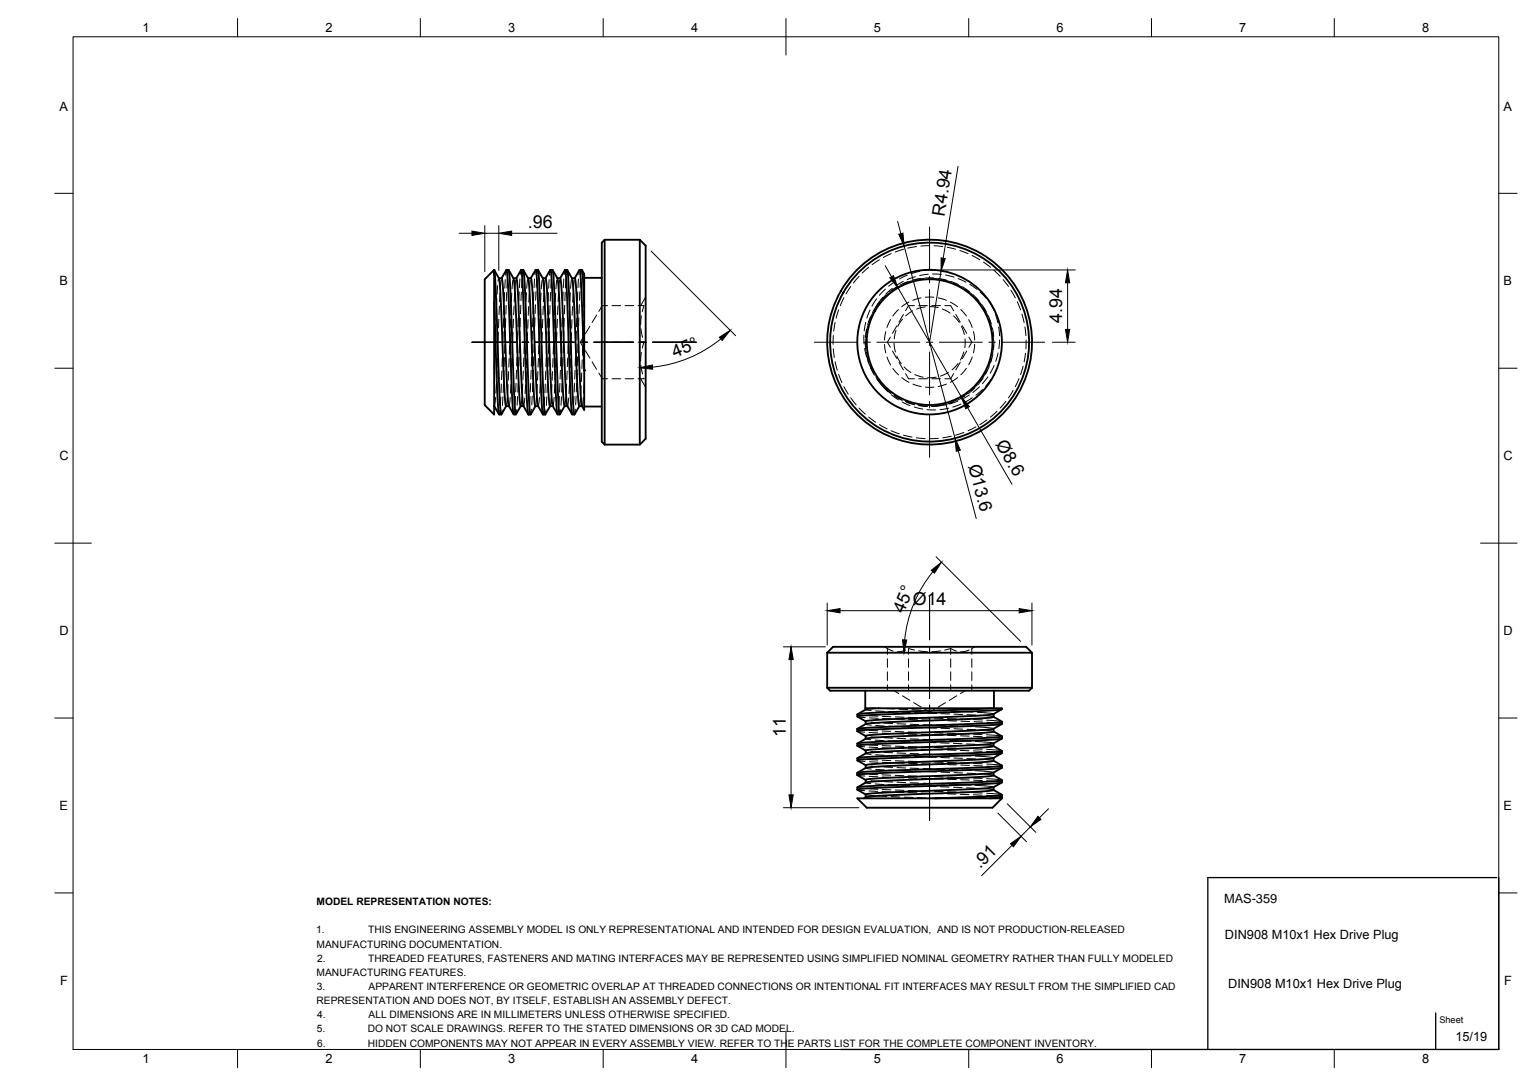
ISO-10303-21;
HEADER;
/* Generated by software containing ST-Developer
 * from STEP Tools, Inc. (www.steptools.com) 
 */

FILE_DESCRIPTION(
/* description */ (''),
/* implementation_level */ '2;1');

FILE_NAME(
/* name */ 'DIN908 M10x1 Hex Drive Plug.step',
/* time_stamp */ '2026-10-15T14:25:16-07:00',
/* author */ (''),
/* organization */ (''),
/* preprocessor_version */ 'ST-DEVELOPER v20.2',
/* originating_system */ 'Autodesk Translation Framework v15.15.0.0',
/* authorisation */ '');

FILE_SCHEMA (('AUTOMOTIVE_DESIGN { 1 0 10303 214 3 1 1 }'));
ENDSEC;

DATA;
#10=MECHANICAL_DESIGN_GEOMETRIC_PRESENTATION_REPRESENTATION('',(#331),#86429);
#254=B_SPLINE_SURFACE_WITH_KNOTS('',3,3,((#65570,#65571,#65572,#65573,#65574,
#65575,#65576,#65577,#65578,#65579,#65580,#65581,#65582,#65583,#65584,#65585,
#65586,#65587,#65588,#65589,#65590,#65591,#65592,#65593,#65594,#65595,#65596,
#65597,#65598,#65599,#65600,#65601,#65602,#65603,#65604,#65605,#65606,#65607,
#65608,#65609,#65610,#65611,#65612,#65613,#65614,#65615),(#65616,#65617,
#65618,#65619,#65620,#65621,#65622,#65623,#65624,#65625,#65626,#65627,#65628,
#65629,#65630,#65631,#65632,#65633,#65634,#65635,#65636,#65637,#65638,#65639,
#65640,#65641,#65642,#65643,#65644,#65645,#65646,#65647,#65648,#65649,#65650,
#65651,#65652,#65653,#65654,#65655,#65656,#65657,#65658,#65659,#65660,#65661),
(#65662,#65663,#65664,#65665,#65666,#65667,#65668,#65669,#65670,#65671,
#65672,#65673,#65674,#65675,#65676,#65677,#65678,#65679,#65680,#65681,#65682,
#65683,#65684,#65685,#65686,#65687,#65688,#65689,#65690,#65691,#65692,#65693,
#65694,#65695,#65696,#65697,#65698,#65699,#65700,#65701,#65702,#65703,#65704,
#65705,#65706,#65707),(#65708,#65709,#65710,#65711,#65712,#65713,#65714,
#65715,#65716,#65717,#65718,#65719,#65720,#65721,#65722,#65723,#65724,#65725,
#65726,#65727,#65728,#65729,#65730,#65731,#65732,#65733,#65734,#65735,#65736,
#65737,#65738,#65739,#65740,#65741,#65742,#65743,#65744,#65745,#65746,#65747,
#65748,#65749,#65750,#65751,#65752,#65753)),.UNSPECIFIED.,.F.,.F.,.F.,(4,
4),(4,1,1,1,1,1,1,1,1,1,1,1,1,1,1,1,1,1,1,1,1,1,1,1,1,1,1,1,1,1,1,1,1,1,
1,1,1,1,1,1,1,1,1,4),(-0.00074044236405861,0.066233565701187),(8.3083844520832,
8.80545257887392,9.30252070566464,10.2966569592461,11.2907932128275,12.284929466409,
13.2790657199904,14.2732019735718,15.2673382271533,16.2614744807347,17.2556107343161,
18.2497469878976,19.243883241479,20.2380194950604,21.2321557486419,22.2262920022233,
23.2204282558048,24.2145645093862,25.2087007629676,26.2028370165491,27.1969732701305,
28.1911095237119,29.1852457772934,30.1793820308748,31.1735182844562,32.1676545380377,
33.1617907916191,34.1559270452005,35.150063298782,36.1441995523634,37.1383358059449,
38.1324720595263,39.1266083131077,40.1207445666892,41.1148808202706,42.109017073852,
43.1031533274335,44.0972895810149,45.0914258345964,46.0855620881778,47.0796983417592,
48.0738345953407,48.5709027221314,49.0687112912862),.UNSPECIFIED.);
#255=B_SPLINE_SURFACE_WITH_KNOTS('',3,3,((#65959,#65960,#65961,#65962,#65963,
#65964,#65965,#65966,#65967,#65968,#65969,#65970,#65971,#65972,#65973,#65974,
#65975,#65976,#65977,#65978,#65979,#65980,#65981,#65982,#65983,#65984,#65985,
#65986,#65987,#65988,#65989,#65990,#65991,#65992,#65993,#65994,#65995,#65996,
#65997,#65998,#65999,#66000,#66001,#66002,#66003,#66004),(#66005,#66006,
#66007,#66008,#66009,#66010,#66011,#66012,#66013,#66014,#66015,#66016,#66017,
#66018,#66019,#66020,#66021,#66022,#66023,#66024,#66025,#66026,#66027,#66028,
#66029,#66030,#66031,#66032,#66033,#66034,#66035,#66036,#66037,#66038,#66039,
#66040,#66041,#66042,#66043,#66044,#66045,#66046,#66047,#66048,#66049,#66050),
(#66051,#66052,#66053,#66054,#66055,#66056,#66057,#66058,#66059,#66060,
#66061,#66062,#66063,#66064,#66065,#66066,#66067,#66068,#66069,#66070,#66071,
#66072,#66073,#66074,#66075,#66076,#66077,#66078,#66079,#66080,#66081,#66082,
#66083,#66084,#66085,#66086,#66087,#66088,#66089,#66090,#66091,#66092,#66093,
#66094,#66095,#66096),(#66097,#66098,#66099,#66100,#66101,#66102,#66103,
#66104,#66105,#66106,#66107,#66108,#66109,#66110,#66111,#66112,#66113,#66114,
#66115,#66116,#66117,#66118,#66119,#66120,#66121,#66122,#66123,#66124,#66125,
#66126,#66127,#66128,#66129,#66130,#66131,#66132,#66133,#66134,#66135,#66136,
#66137,#66138,#66139,#66140,#66141,#66142)),.UNSPECIFIED.,.F.,.F.,.F.,(4,
4),(4,1,1,1,1,1,1,1,1,1,1,1,1,1,1,1,1,1,1,1,1,1,1,1,1,1,1,1,1,1,1,1,1,1,
1,1,1,1,1,1,1,1,1,4),(-0.000415672852192788,0.0663202636511997),(11.6148054166941,
12.112100974609,12.6091691013998,13.6033053549812,14.5974416085626,15.5915778621441,
16.5857141157255,17.5798503693069,18.5739866228884,19.5681228764698,20.5622591300512,
21.5563953836327,22.5505316372141,23.5446678907956,24.538804144377,25.5329403979584,
26.5270766515399,27.5212129051213,28.5153491587027,29.5094854122842,30.5036216658656,
31.497757919447,32.4918941730285,33.4860304266099,34.4801666801914,35.4743029337728,
36.4684391873542,37.4625754409357,38.4567116945171,39.4508479480985,40.44498420168,
41.4391204552614,42.4332567088428,43.4273929624243,44.4215292160057,45.4156654695872,
46.4098017231686,47.40393797675,48.3980742303315,49.3922104839129,50.3863467374943,
51.3804829910758,51.8775511178665,52.3746192446572),.UNSPECIFIED.);
#266=(
BOUNDED_CURVE()
B_SPLINE_CURVE(2,(#66219,#66220,#66221),.UNSPECIFIED.,.F.,.F.)
B_SPLINE_CURVE_WITH_KNOTS((3,3),(-0.639366558443437,-0.433164349146202),
 .UNSPECIFIED.)
CURVE()
GEOMETRIC_REPRESENTATION_ITEM()
RATIONAL_B_SPLINE_CURVE((1.35866716012837,1.4637604307034,1.4637604307034))
REPRESENTATION_ITEM('')
);
#267=(
BOUNDED_CURVE()
B_SPLINE_CURVE(2,(#66223,#66224,#66225),.UNSPECIFIED.,.F.,.F.)
B_SPLINE_CURVE_WITH_KNOTS((3,3),(0.0319010196424348,0.336489692457453),
 .UNSPECIFIED.)
CURVE()
GEOMETRIC_REPRESENTATION_ITEM()
RATIONAL_B_SPLINE_CURVE((1.03712812921102,1.19757240916823,1.03712812921102))
REPRESENTATION_ITEM('')
);
#268=(
BOUNDED_CURVE()
B_SPLINE_CURVE(2,(#66227,#66228,#66229),.UNSPECIFIED.,.F.,.F.)
B_SPLINE_CURVE_WITH_KNOTS((3,3),(0.0319010196424347,0.336489692457453),
 .UNSPECIFIED.)
CURVE()
GEOMETRIC_REPRESENTATION_ITEM()
RATIONAL_B_SPLINE_CURVE((1.03712812921102,1.19757240916823,1.03712812921102))
REPRESENTATION_ITEM('')
);
#269=(
BOUNDED_CURVE()
B_SPLINE_CURVE(2,(#66231,#66232,#66233),.UNSPECIFIED.,.F.,.F.)
B_SPLINE_CURVE_WITH_KNOTS((3,3),(0.0319010196424348,0.336489692457453),
 .UNSPECIFIED.)
CURVE()
GEOMETRIC_REPRESENTATION_ITEM()
RATIONAL_B_SPLINE_CURVE((1.03712812921102,1.19757240916823,1.03712812921102))
REPRESENTATION_ITEM('')
);
#270=(
BOUNDED_CURVE()
B_SPLINE_CURVE(2,(#66235,#66236,#66237),.UNSPECIFIED.,.F.,.F.)
B_SPLINE_CURVE_WITH_KNOTS((3,3),(0.0319010196424349,0.336489692457453),
 .UNSPECIFIED.)
CURVE()
GEOMETRIC_REPRESENTATION_ITEM()
RATIONAL_B_SPLINE_CURVE((1.03712812921102,1.19757240916823,1.03712812921102))
REPRESENTATION_ITEM('')
);
#271=(
BOUNDED_CURVE()
B_SPLINE_CURVE(2,(#66239,#66240,#66241),.UNSPECIFIED.,.F.,.F.)
B_SPLINE_CURVE_WITH_KNOTS((3,3),(0.0319010196424347,0.336489692457453),
 .UNSPECIFIED.)
CURVE()
GEOMETRIC_REPRESENTATION_ITEM()
RATIONAL_B_SPLINE_CURVE((1.03712812921102,1.19757240916823,1.03712812921102))
REPRESENTATION_ITEM('')
);
#272=(
BOUNDED_CURVE()
B_SPLINE_CURVE(2,(#66242,#66243,#66244),.UNSPECIFIED.,.F.,.F.)
B_SPLINE_CURVE_WITH_KNOTS((3,3),(-0.433164349146202,-0.226962139848967),
 .UNSPECIFIED.)
CURVE()
GEOMETRIC_REPRESENTATION_ITEM()
RATIONAL_B_SPLINE_CURVE((1.4637604307034,1.4637604307034,1.35866716012837))
REPRESENTATION_ITEM('')
);
#295=SHAPE_REPRESENTATION_RELATIONSHIP('SRR','None',#86510,#313);
#313=ADVANCED_BREP_SHAPE_REPRESENTATION('',(#349),#86419);
#331=STYLED_ITEM('',(#86609),#349);
#349=MANIFOLD_SOLID_BREP('Body1',#15621);
#898=B_SPLINE_CURVE_WITH_KNOTS('',3,(#63261,#63262,#63263,#63264,#63265,
#63266,#63267,#63268,#63269,#63270,#63271,#63272,#63273,#63274,#63275,#63276,
#63277,#63278,#63279,#63280,#63281,#63282,#63283,#63284,#63285,#63286,#63287,
#63288,#63289,#63290,#63291,#63292,#63293,#63294,#63295,#63296,#63297,#63298,
#63299,#63300,#63301,#63302,#63303,#63304,#63305,#63306,#63307,#63308,#63309,
#63310,#63311,#63312,#63313,#63314,#63315,#63316,#63317,#63318,#63319,#63320,
#63321,#63322,#63323,#63324,#63325,#63326,#63327,#63328,#63329,#63330,#63331,
#63332,#63333,#63334,#63335,#63336,#63337,#63338,#63339),.UNSPECIFIED.,
 .F.,.F.,(4,3,3,3,3,3,3,3,3,3,3,3,3,3,3,3,3,3,3,3,3,3,3,3,3,3,4),(10.3769577827544,
10.5273598900866,10.6774945443399,10.8308192114618,10.9808890436316,11.1358411282296,
11.2907932128275,11.4445181516619,11.5979719285541,11.7512647292242,11.9046292861554,
12.0580308496751,12.211755396569,12.284929466409,12.4385133838143,12.5918292435621,
12.7449877126714,12.8982250015488,13.0515031898628,13.2051123582851,13.2790657199904,
13.432297699739,13.5852451018772,13.7380996304701,13.8908875290217,14.0438933465584,
14.1577916878073),.UNSPECIFIED.);
#899=B_SPLINE_CURVE_WITH_KNOTS('',3,(#63342,#63343,#63344,#63345,#63346,
#63347,#63348,#63349,#63350,#63351,#63352,#63353,#63354,#63355,#63356,#63357,
#63358,#63359,#63360,#63361,#63362,#63363,#63364,#63365,#63366,#63367,#63368,
#63369,#63370,#63371,#63372,#63373,#63374,#63375,#63376,#63377,#63378,#63379,
#63380,#63381,#63382,#63383,#63384,#63385,#63386,#63387,#63388,#63389,#63390,
#63391,#63392,#63393,#63394,#63395,#63396),.UNSPECIFIED.,.F.,.F.,(4,3,3,
3,3,3,3,3,3,3,3,3,3,3,3,3,3,3,4),(11.6150328478183,11.7926764189461,11.9701488858192,
12.112100974609,12.2661530434337,12.4201862996183,12.5744137841679,12.6091691013998,
12.7645204088578,12.919681016886,13.0747528344925,13.2299786470436,13.3852896170894,
13.5409644760237,13.6033053549812,13.7553480979553,13.9070954748021,14.0586995150233,
14.1583240782391),.UNSPECIFIED.);
#900=B_SPLINE_CURVE_WITH_KNOTS('',3,(#63402,#63403,#63404,#63405,#63406,
#63407,#63408,#63409,#63410,#63411,#63412,#63413,#63414,#63415,#63416,#63417,
#63418,#63419,#63420,#63421,#63422,#63423,#63424,#63425,#63426,#63427,#63428,
#63429,#63430,#63431,#63432,#63433,#63434,#63435,#63436,#63437,#63438,#63439,
#63440,#63441,#63442,#63443,#63444,#63445,#63446,#63447,#63448,#63449,#63450,
#63451,#63452,#63453,#63454,#63455,#63456,#63457,#63458,#63459,#63460,#63461,
#63462,#63463,#63464,#63465,#63466,#63467,#63468,#63469,#63470,#63471,#63472,
#63473,#63474,#63475,#63476,#63477,#63478,#63479,#63480,#63481,#63482,#63483,
#63484,#63485,#63486,#63487,#63488,#63489,#63490,#63491,#63492,#63493,#63494,
#63495,#63496,#63497,#63498,#63499,#63500,#63501,#63502,#63503,#63504),
 .UNSPECIFIED.,.F.,.F.,(4,3,3,3,3,3,3,3,3,3,3,3,3,3,3,3,3,3,3,3,3,3,3,3,
3,3,3,3,3,3,3,3,3,3,4),(15.7079632679489,15.8650809592317,16.0223560154779,
16.180095481684,16.2614744807347,16.414856728946,16.5679648062975,16.7209100993148,
16.8739286197668,17.0269845627285,17.1803695780412,17.2556107343161,17.4090275970834,
17.5621709487349,17.7151520567367,17.8682067844267,18.021299206932,18.1747205540646,
18.2497469878976,18.4031557793674,18.5562910052633,18.7092639603358,18.8623105909142,
19.0153949374731,19.1688083680783,19.243883241479,19.3972872546799,19.5504175546535,
19.703385452925,19.8564268889446,20.0095059553496,20.1629140554059,20.2380194950604,
20.3914408227308,20.4420478592521),.UNSPECIFIED.);
#901=B_SPLINE_CURVE_WITH_KNOTS('',3,(#63505,#63506,#63507,#63508,#63509,
#63510,#63511,#63512,#63513,#63514,#63515,#63516,#63517,#63518,#63519,#63520,
#63521,#63522,#63523,#63524,#63525,#63526,#63527,#63528,#63529,#63530,#63531,
#63532,#63533,#63534,#63535,#63536,#63537,#63538),.UNSPECIFIED.,.F.,.F.,
(4,3,3,3,3,3,3,3,3,3,3,4),(14.1577916878073,14.2732019735718,14.4266654812486,
14.5798559651052,14.7328845330507,14.8859866502668,15.039126483985,15.1925945327221,
15.2673382271533,15.4330590962838,15.5979020456747,15.7079632678343),
 .UNSPECIFIED.);
#902=B_SPLINE_CURVE_WITH_KNOTS('',3,(#63540,#63541,#63542,#63543,#63544,
#63545,#63546,#63547,#63548,#63549,#63550,#63551,#63552,#63553,#63554,#63555,
#63556,#63557,#63558,#63559,#63560,#63561,#63562,#63563,#63564,#63565,#63566,
#63567,#63568,#63569,#63570,#63571,#63572,#63573),.UNSPECIFIED.,.F.,.F.,
(4,3,3,3,3,3,3,3,3,3,3,4),(14.1583240782391,14.3099489598577,14.4619231331325,
14.5974416085626,14.7511673052192,14.9046218555822,15.05791544251,15.2112807951612,
15.3646831606929,15.5184085065351,15.5915778621441,15.707963267949),
 .UNSPECIFIED.);
#903=B_SPLINE_CURVE_WITH_KNOTS('',3,(#63574,#63575,#63576,#63577,#63578,
#63579,#63580,#63581,#63582,#63583,#63584,#63585,#63586,#63587,#63588,#63589,
#63590,#63591,#63592,#63593,#63594,#63595,#63596,#63597,#63598,#63599,#63600,
#63601,#63602,#63603,#63604,#63605,#63606,#63607,#63608,#63609,#63610,#63611,
#63612,#63613,#63614,#63615,#63616,#63617,#63618,#63619,#63620,#63621,#63622,
#63623,#63624,#63625,#63626,#63627,#63628,#63629,#63630,#63631,#63632,#63633,
#63634,#63635,#63636,#63637,#63638,#63639,#63640,#63641,#63642,#63643,#63644,
#63645,#63646,#63647,#63648,#63649,#63650,#63651,#63652,#63653,#63654,#63655,
#63656,#63657,#63658,#63659,#63660,#63661,#63662,#63663,#63664,#63665,#63666,
#63667,#63668,#63669,#63670,#63671,#63672,#63673),.UNSPECIFIED.,.F.,.F.,
(4,3,3,3,3,3,3,3,3,3,3,3,3,3,3,3,3,3,3,3,3,3,3,3,3,3,3,3,3,3,3,3,3,4),(15.7079632680668,
15.8594388736004,16.0106884436182,16.1619521092882,16.3132060736808,16.4647924609641,
16.5857141157255,16.7389389348221,16.8918864719011,17.0446686448837,17.1975220592675,
17.3504115327853,17.5036305542145,17.5798503693069,17.733313923022,17.886504454532,
18.0395330715724,18.1926352394518,18.3457751247938,18.4992432258178,18.5739866228884,
18.7274115805076,18.8805635511898,19.033553772357,19.1866182515782,19.3397208031865,
19.4931527076817,19.5681228764698,19.7215125444031,19.8746204229269,20.0276355842012,
20.1805858124463,20.3337471975624,20.4409723240163),.UNSPECIFIED.);
#904=B_SPLINE_CURVE_WITH_KNOTS('',3,(#63679,#63680,#63681,#63682,#63683,
#63684,#63685,#63686,#63687,#63688,#63689,#63690,#63691,#63692,#63693,#63694,
#63695,#63696,#63697,#63698,#63699,#63700,#63701,#63702,#63703,#63704,#63705,
#63706,#63707,#63708,#63709,#63710,#63711,#63712,#63713,#63714,#63715,#63716,
#63717,#63718,#63719,#63720,#63721,#63722,#63723,#63724,#63725,#63726,#63727,
#63728,#63729,#63730,#63731,#63732,#63733,#63734,#63735,#63736,#63737,#63738,
#63739,#63740,#63741,#63742,#63743,#63744,#63745,#63746,#63747,#63748,#63749,
#63750,#63751,#63752,#63753,#63754,#63755,#63756,#63757,#63758,#63759,#63760,
#63761,#63762,#63763,#63764,#63765,#63766,#63767,#63768,#63769,#63770,#63771,
#63772,#63773,#63774,#63775,#63776,#63777,#63778,#63779,#63780,#63781),
 .UNSPECIFIED.,.F.,.F.,(4,3,3,3,3,3,3,3,3,3,3,3,3,3,3,3,3,3,3,3,3,3,3,3,
3,3,3,3,3,3,3,3,3,3,4),(21.99114857526,22.1939267919493,22.2262920022233,
22.3796989418416,22.5328322331403,22.6858031775158,22.838847706263,22.9919298961389,
23.145341118553,23.2204282558048,23.3738358680276,23.5269698461768,23.6799414893234,
23.8329867265599,23.9860696314175,24.13948156771,24.2145645093862,24.3679718714795,
24.5211055961752,24.6740769833984,24.827121964018,24.9802046115219,25.1336162933461,
25.2087007629676,25.3621080840594,25.5152417657962,25.6682131082504,25.8212580418961,
25.9743406411039,26.127752273332,26.2028370165491,26.3562428141984,26.5093760788686,
26.662367028694,26.7245753429587),.UNSPECIFIED.);
#905=B_SPLINE_CURVE_WITH_KNOTS('',3,(#63782,#63783,#63784,#63785,#63786,
#63787,#63788,#63789,#63790,#63791,#63792,#63793,#63794,#63795,#63796,#63797,
#63798,#63799,#63800,#63801,#63802,#63803,#63804,#63805,#63806,#63807,#63808,
#63809,#63810,#63811,#63812,#63813,#63814,#63815),.UNSPECIFIED.,.F.,.F.,
(4,3,3,3,3,3,3,3,3,3,3,4),(20.4420478592521,20.5951172325546,20.7543768615764,
20.9074258209389,21.0605493555233,21.2139862899396,21.2321557486419,21.3836611788031,
21.5355330278844,21.6866431849307,21.8388958800296,21.9911485751285),
 .UNSPECIFIED.);
#906=B_SPLINE_CURVE_WITH_KNOTS('',3,(#63817,#63818,#63819,#63820,#63821,
#63822,#63823,#63824,#63825,#63826,#63827,#63828,#63829,#63830,#63831,#63832,
#63833,#63834,#63835,#63836,#63837,#63838,#63839,#63840,#63841,#63842,#63843,
#63844,#63845,#63846,#63847,#63848,#63849,#63850),.UNSPECIFIED.,.F.,.F.,
(4,3,3,3,3,3,3,3,3,3,3,4),(20.4409723240163,20.5622591300512,20.7156759866491,
20.8688193321945,21.0218004341724,21.1748551560304,21.3279475728055,21.4813689144523,
21.5563953836327,21.7227148730573,21.8881132512756,21.9911485750061),
 .UNSPECIFIED.);
#907=B_SPLINE_CURVE_WITH_KNOTS('',3,(#63851,#63852,#63853,#63854,#63855,
#63856,#63857,#63858,#63859,#63860,#63861,#63862,#63863,#63864,#63865,#63866,
#63867,#63868,#63869,#63870,#63871,#63872,#63873,#63874,#63875,#63876,#63877,
#63878,#63879,#63880,#63881,#63882,#63883,#63884,#63885,#63886,#63887,#63888,
#63889,#63890,#63891,#63892,#63893,#63894,#63895,#63896,#63897,#63898,#63899,
#63900,#63901,#63902,#63903,#63904,#63905,#63906,#63907,#63908,#63909,#63910,
#63911,#63912,#63913,#63914,#63915,#63916,#63917,#63918,#63919,#63920,#63921,
#63922,#63923,#63924,#63925,#63926,#63927,#63928,#63929,#63930,#63931,#63932,
#63933,#63934,#63935,#63936,#63937,#63938,#63939,#63940,#63941,#63942,#63943,
#63944,#63945,#63946,#63947,#63948,#63949,#63950,#63951,#63952,#63953),
 .UNSPECIFIED.,.F.,.F.,(4,3,3,3,3,3,3,3,3,3,3,3,3,3,3,3,3,3,3,3,3,3,3,3,
3,3,3,3,3,3,3,3,3,3,4),(21.9911485751285,22.1479256648879,22.3048452391874,
22.462221546967,22.5505316372141,22.703935658999,22.8570659677062,23.0100338748324,
23.1630753197854,23.3161543951809,23.469562504177,23.5446678907956,23.6980767887443,
23.8512120717938,24.0041850346144,24.1572315981784,24.3103158349244,24.4637290908905,
24.538804144377,24.6922115651092,24.8453453550659,24.9983168139393,25.1513618750143,
25.3044446081105,25.4578563821735,25.5329403979584,25.6863473392698,25.8394806322957,
25.9924515784266,26.145496108951,26.2985783006192,26.4519895248209,26.5270766515399,
26.6804991039507,26.7252324446079),.UNSPECIFIED.);
#908=B_SPLINE_CURVE_WITH_KNOTS('',3,(#63959,#63960,#63961,#63962,#63963,
#63964,#63965,#63966,#63967,#63968,#63969,#63970,#63971,#63972,#63973,#63974,
#63975,#63976,#63977,#63978,#63979,#63980,#63981,#63982,#63983,#63984,#63985,
#63986,#63987,#63988,#63989,#63990,#63991,#63992,#63993,#63994,#63995,#63996,
#63997,#63998,#63999,#64000,#64001,#64002,#64003,#64004,#64005,#64006,#64007,
#64008,#64009,#64010,#64011,#64012,#64013,#64014,#64015,#64016,#64017,#64018,
#64019,#64020,#64021,#64022,#64023,#64024,#64025,#64026,#64027,#64028,#64029,
#64030,#64031,#64032,#64033,#64034,#64035,#64036,#64037,#64038,#64039,#64040,
#64041,#64042,#64043,#64044,#64045,#64046,#64047,#64048,#64049,#64050,#64051,
#64052,#64053,#64054,#64055,#64056,#64057,#64058),.UNSPECIFIED.,.F.,.F.,
(4,3,3,3,3,3,3,3,3,3,3,3,3,3,3,3,3,3,3,3,3,3,3,3,3,3,3,3,3,3,3,3,3,4),(28.2743338824354,
28.4259808413042,28.5773785225841,28.7293453362614,28.8807048174512,29.0329752973723,
29.1852457772934,29.3386531544532,29.4917868936077,29.644758294636,29.7978032879121,
29.9508859474332,30.104297640095,30.1793820308748,30.3327894432698,30.4859232177876,
30.6388946541924,30.7919396824536,30.9450223767831,31.0984341034409,31.1735182844562,
31.3269256011464,31.480059280071,31.6330306212942,31.7860755560757,31.9391581577712,
32.0925697945182,32.1676545380377,32.3210720983193,32.4742063232938,32.6272330512433,
32.7801943527862,32.9333288292476,33.0072870494089),.UNSPECIFIED.);
#909=B_SPLINE_CURVE_WITH_KNOTS('',3,(#64059,#64060,#64061,#64062,#64063,
#64064,#64065,#64066,#64067,#64068,#64069,#64070,#64071,#64072,#64073,#64074,
#64075,#64076,#64077,#64078,#64079,#64080,#64081,#64082,#64083,#64084,#64085,
#64086,#64087,#64088,#64089,#64090,#64091,#64092),.UNSPECIFIED.,.F.,.F.,
(4,3,3,3,3,3,3,3,3,3,3,4),(26.7245753429587,26.8776236986561,27.0372984843933,
27.1969732701305,27.3503806471368,27.5035143861932,27.6564857871786,27.8095307804943,
27.9626134401022,28.1160251329216,28.1911095237119,28.2743338823081),
 .UNSPECIFIED.);
#910=B_SPLINE_CURVE_WITH_KNOTS('',3,(#64094,#64095,#64096,#64097,#64098,
#64099,#64100,#64101,#64102,#64103,#64104,#64105,#64106,#64107,#64108,#64109,
#64110,#64111,#64112,#64113,#64114,#64115,#64116,#64117,#64118,#64119,#64120,
#64121,#64122,#64123,#64124,#64125,#64126,#64127),.UNSPECIFIED.,.F.,.F.,
(4,3,3,3,3,3,3,3,3,3,3,4),(26.7252324446079,26.8783075285994,27.0390338727299,
27.1920808254545,27.3451994950597,27.498632670491,27.5212129051213,27.672785837319,
27.8241164256345,27.9752896314244,28.1265899278275,28.2743338823081),
 .UNSPECIFIED.);
#911=B_SPLINE_CURVE_WITH_KNOTS('',3,(#64128,#64129,#64130,#64131,#64132,
#64133,#64134,#64135,#64136,#64137,#64138,#64139,#64140,#64141,#64142,#64143,
#64144,#64145,#64146,#64147,#64148,#64149,#64150,#64151,#64152,#64153,#64154,
#64155,#64156,#64157,#64158,#64159,#64160,#64161,#64162,#64163,#64164,#64165,
#64166,#64167,#64168,#64169,#64170,#64171,#64172,#64173,#64174,#64175,#64176,
#64177,#64178,#64179,#64180,#64181,#64182,#64183,#64184,#64185,#64186,#64187,
#64188,#64189,#64190,#64191,#64192,#64193,#64194,#64195,#64196,#64197,#64198,
#64199,#64200,#64201,#64202,#64203,#64204,#64205,#64206,#64207,#64208,#64209,
#64210,#64211,#64212,#64213,#64214,#64215,#64216,#64217,#64218,#64219,#64220,
#64221,#64222,#64223,#64224,#64225,#64226,#64227,#64228,#64229,#64230),
 .UNSPECIFIED.,.F.,.F.,(4,3,3,3,3,3,3,3,3,3,3,3,3,3,3,3,3,3,3,3,3,3,3,3,
3,3,3,3,3,3,3,3,3,3,4),(28.2743338824879,28.4750398536421,28.5153491587027,
28.6687564800878,28.8218901621242,28.9748615048833,29.1279064388382,29.2809890383584,
29.4344006708985,29.5094854122842,29.6628928231069,29.8160265965599,29.9689980324053,
30.1220430608655,30.2751257558269,30.4285374837698,30.5036216658656,30.6570290428525,
30.810162781889,30.9631341828541,31.1161791761489,31.2692618357356,31.4226735285337,
31.497757919447,31.651165282527,31.8042990074916,31.9572703942643,32.1103153733462,
32.2633980186889,32.4168096974117,32.4918941730285,32.6453002476881,32.7984336411736,
32.9514213448994,33.0077784099125),.UNSPECIFIED.);
#912=B_SPLINE_CURVE_WITH_KNOTS('',3,(#64236,#64237,#64238,#64239,#64240,
#64241,#64242,#64243,#64244,#64245,#64246,#64247,#64248,#64249,#64250,#64251,
#64252,#64253,#64254,#64255,#64256,#64257,#64258,#64259,#64260,#64261,#64262,
#64263,#64264,#64265,#64266,#64267,#64268,#64269,#64270,#64271,#64272,#64273,
#64274,#64275,#64276,#64277,#64278,#64279,#64280,#64281,#64282,#64283,#64284,
#64285,#64286,#64287,#64288,#64289,#64290,#64291,#64292,#64293,#64294,#64295,
#64296,#64297,#64298,#64299,#64300,#64301,#64302,#64303,#64304,#64305,#64306,
#64307,#64308,#64309,#64310,#64311,#64312,#64313,#64314,#64315,#64316,#64317,
#64318,#64319,#64320,#64321,#64322,#64323,#64324,#64325,#64326,#64327,#64328,
#64329,#64330,#64331,#64332,#64333,#64334,#64335,#64336,#64337,#64338),
 .UNSPECIFIED.,.F.,.F.,(4,3,3,3,3,3,3,3,3,3,3,3,3,3,3,3,3,3,3,3,3,3,3,3,
3,3,3,3,3,3,3,3,3,3,4),(34.5575191894877,34.7128109395726,34.8681775956844,
35.0239713658574,35.150063298782,35.3034707576981,35.456604572422,35.6095760427116,
35.762621095208,35.915703808308,36.0691155452003,36.1441995523634,36.2976084936062,
36.4507438054633,36.6037167826695,36.7567633389953,36.9098475561584,37.0632607739405,
37.1383358059449,37.291739596941,37.4448697549461,37.5978375910733,37.7508790844318,
37.9039582764099,38.0573666045902,38.1324720595263,38.2858811685694,38.4390165973614,
38.5919896412426,38.745036189863,38.8981203569408,39.0515334615024,39.1266083131077,
39.2800571769567,39.2915821620202),.UNSPECIFIED.);
#913=B_SPLINE_CURVE_WITH_KNOTS('',3,(#64339,#64340,#64341,#64342,#64343,
#64344,#64345,#64346,#64347,#64348,#64349,#64350,#64351,#64352,#64353,#64354,
#64355,#64356,#64357,#64358,#64359,#64360,#64361,#64362,#64363,#64364,#64365,
#64366,#64367,#64368,#64369,#64370,#64371,#64372),.UNSPECIFIED.,.F.,.F.,
(4,3,3,3,3,3,3,3,3,3,3,4),(33.0072870494089,33.1617907916191,33.3151984118971,
33.4683323951928,33.6213040405922,33.77434927575,33.9274321760551,34.0808441040777,
34.1559270452005,34.3257930361133,34.4944769778812,34.5575191893185),
 .UNSPECIFIED.);
#914=B_SPLINE_CURVE_WITH_KNOTS('',3,(#64374,#64375,#64376,#64377,#64378,
#64379,#64380,#64381,#64382,#64383,#64384,#64385,#64386,#64387,#64388,#64389,
#64390,#64391,#64392,#64393,#64394,#64395,#64396,#64397,#64398,#64399,#64400,
#64401,#64402,#64403,#64404,#64405,#64406,#64407,#64408,#64409,#64410),
 .UNSPECIFIED.,.F.,.F.,(4,3,3,3,3,3,3,3,3,3,3,3,4),(33.0077784099125,33.1608257171148,
33.3139472904311,33.4673823924497,33.4860304266099,33.6394378388404,33.7925716131929,
33.9455430494321,34.098588077529,34.2516707716947,34.4050824981922,34.4801666801914,
34.5575191894877),.UNSPECIFIED.);
#915=B_SPLINE_CURVE_WITH_KNOTS('',3,(#64411,#64412,#64413,#64414,#64415,
#64416,#64417,#64418,#64419,#64420,#64421,#64422,#64423,#64424,#64425,#64426,
#64427,#64428,#64429,#64430,#64431,#64432,#64433,#64434,#64435,#64436,#64437,
#64438,#64439,#64440,#64441,#64442,#64443,#64444,#64445,#64446,#64447,#64448,
#64449,#64450,#64451,#64452,#64453,#64454,#64455,#64456,#64457,#64458,#64459,
#64460,#64461,#64462,#64463,#64464,#64465,#64466,#64467,#64468,#64469,#64470,
#64471,#64472,#64473,#64474,#64475,#64476,#64477,#64478,#64479,#64480,#64481,
#64482,#64483,#64484,#64485,#64486,#64487,#64488,#64489,#64490,#64491,#64492,
#64493,#64494,#64495,#64496,#64497,#64498,#64499,#64500,#64501,#64502,#64503,
#64504,#64505,#64506,#64507,#64508,#64509,#64510),.UNSPECIFIED.,.F.,.F.,
(4,3,3,3,3,3,3,3,3,3,3,3,3,3,3,3,3,3,3,3,3,3,3,3,3,3,3,3,3,3,3,3,3,4),(34.5575191896116,
34.7092547626843,34.8607382426211,35.014129415409,35.165569538894,35.3199362363334,
35.4743029337728,35.6277102998244,35.7808440270258,35.9338154153095,36.0868603948273,
36.2399430399945,36.3933547176269,36.4684391873542,36.6218468068268,36.7749807893111,
36.9279524338957,37.0809976682432,37.2340805677396,37.3874924949681,37.4625754409357,
37.6159823503777,37.7691156230423,37.9220865602605,38.0751310990094,38.2282133086885,
38.3816245656092,38.4567116945171,38.610129889132,38.7632643739221,38.916288756662,
39.0692475637796,39.2223732435226,39.2904651979605),.UNSPECIFIED.);
#916=B_SPLINE_CURVE_WITH_KNOTS('',3,(#64516,#64517,#64518,#64519,#64520,
#64521,#64522,#64523,#64524,#64525,#64526,#64527,#64528,#64529,#64530,#64531,
#64532,#64533,#64534,#64535,#64536,#64537,#64538,#64539,#64540,#64541,#64542,
#64543,#64544,#64545,#64546,#64547,#64548,#64549,#64550,#64551,#64552,#64553,
#64554,#64555,#64556,#64557,#64558,#64559,#64560,#64561,#64562,#64563,#64564,
#64565,#64566,#64567,#64568,#64569,#64570,#64571,#64572,#64573,#64574,#64575,
#64576,#64577,#64578,#64579,#64580,#64581,#64582,#64583,#64584,#64585,#64586,
#64587,#64588,#64589,#64590,#64591,#64592,#64593,#64594,#64595,#64596,#64597,
#64598,#64599,#64600,#64601,#64602,#64603,#64604,#64605,#64606,#64607,#64608,
#64609,#64610,#64611,#64612,#64613,#64614,#64615,#64616,#64617,#64618),
 .UNSPECIFIED.,.F.,.F.,(4,3,3,3,3,3,3,3,3,3,3,3,3,3,3,3,3,3,3,3,3,3,3,3,
3,3,3,3,3,3,3,3,3,3,4),(40.840704496861,41.0315513197139,41.1148808202706,
41.2683084070192,41.4214620763041,41.5744530701636,41.727516935667,41.8806180818076,
42.0340473903573,42.109017073852,42.2624807464789,42.4156713357008,42.5686999497321,
42.7218020243238,42.8749417647447,43.0284096440709,43.1031533274335,43.256368374023,
43.4093096679249,43.5620891086826,43.714945049858,43.8678400512264,44.021069118693,
44.0972895810149,44.2508939544776,44.404222874785,44.5573870466767,44.7106190333205,
44.8638856297818,45.0174737708723,45.0914258345964,45.2451470488387,45.3985988150857,
45.5518916188261,45.5743044775645),.UNSPECIFIED.);
#917=B_SPLINE_CURVE_WITH_KNOTS('',3,(#64619,#64620,#64621,#64622,#64623,
#64624,#64625,#64626,#64627,#64628,#64629,#64630,#64631,#64632,#64633,#64634,
#64635,#64636,#64637,#64638,#64639,#64640,#64641,#64642,#64643,#64644,#64645,
#64646,#64647,#64648,#64649,#64650,#64651,#64652),.UNSPECIFIED.,.F.,.F.,
(4,3,3,3,3,3,3,3,3,3,3,4),(39.2915821620202,39.4447095027457,39.5976829127759,
39.7507369759808,39.9038361708233,40.0572607936133,40.1207445666892,40.2727807639225,
40.4245502282633,40.5761563774086,40.7278367229112,40.8407044966673),
 .UNSPECIFIED.);
#918=B_SPLINE_CURVE_WITH_KNOTS('',3,(#64654,#64655,#64656,#64657,#64658,
#64659,#64660,#64661,#64662,#64663,#64664,#64665,#64666,#64667,#64668,#64669,
#64670,#64671,#64672,#64673,#64674,#64675,#64676,#64677,#64678,#64679,#64680,
#64681,#64682,#64683,#64684,#64685,#64686,#64687),.UNSPECIFIED.,.F.,.F.,
(4,3,3,3,3,3,3,3,3,3,3,4),(39.2904651979605,39.4508479480985,39.6042568862644,
39.7573921950086,39.910365169076,40.0634117222608,40.2164959362774,40.3699091509537,
40.44498420168,40.6155411212441,40.7848606623605,40.8407044964945),
 .UNSPECIFIED.);
#919=B_SPLINE_CURVE_WITH_KNOTS('',3,(#64688,#64689,#64690,#64691,#64692,
#64693,#64694,#64695,#64696,#64697,#64698,#64699,#64700,#64701,#64702,#64703,
#64704,#64705,#64706,#64707,#64708,#64709,#64710,#64711,#64712,#64713,#64714,
#64715,#64716,#64717,#64718,#64719,#64720,#64721,#64722,#64723,#64724,#64725,
#64726,#64727,#64728,#64729,#64730,#64731,#64732,#64733,#64734,#64735,#64736,
#64737,#64738,#64739,#64740,#64741,#64742,#64743,#64744,#64745,#64746,#64747,
#64748,#64749,#64750,#64751,#64752,#64753,#64754,#64755,#64756,#64757,#64758,
#64759,#64760,#64761,#64762,#64763,#64764,#64765,#64766,#64767,#64768,#64769,
#64770,#64771,#64772,#64773,#64774,#64775,#64776,#64777,#64778,#64779,#64780,
#64781,#64782,#64783,#64784,#64785,#64786,#64787),.UNSPECIFIED.,.F.,.F.,
(4,3,3,3,3,3,3,3,3,3,3,3,3,3,3,3,3,3,3,3,3,3,3,3,3,3,3,3,3,3,3,3,3,4),(40.8407044966673,
40.9957591292645,41.1508780734467,41.3064201957631,41.4391204552614,41.5925295553931,
41.7456649753238,41.8986380104205,42.0516845504698,42.2047687090867,42.3581818054854,
42.4332567088428,42.5866737227815,42.7398171688485,42.8927983148208,43.0458529960652,
43.1989453239065,43.3523665040073,43.4273929624243,43.5807737407789,43.7338808906567,
43.8868257956909,44.0398447353975,44.19290155861,44.3462881466742,44.4215292160057,
44.5749567504601,44.7281103673692,44.8811013089363,45.0341651228667,45.1872662177759,
45.3406954764042,45.4156654695872,45.5747633669549),.UNSPECIFIED.);
#920=B_SPLINE_CURVE_WITH_KNOTS('',3,(#64791,#64792,#64793,#64794,#64795,
#64796,#64797,#64798,#64799,#64800,#64801,#64802,#64803,#64804,#64805,#64806,
#64807,#64808,#64809,#64810,#64811,#64812,#64813,#64814,#64815,#64816,#64817,
#64818,#64819,#64820,#64821,#64822,#64823,#64824,#64825,#64826,#64827,#64828,
#64829,#64830,#64831,#64832,#64833,#64834,#64835,#64836),.UNSPECIFIED.,
 .F.,.F.,(4,3,3,3,3,3,3,3,3,3,3,3,3,3,3,4),(-4.09293042013064,-3.97654501432575,
-3.82746242150663,-3.67863474659495,-3.5299614831974,-3.38122102744219,
-3.23245410916824,-3.08336698099754,-2.98240876074431,-2.83653578429899,
-2.69091995422318,-2.54545308154322,-2.39991629923551,-2.25433443827349,
-2.10845930416463,-2.06815232264671),.UNSPECIFIED.);
#921=B_SPLINE_CURVE_WITH_KNOTS('',3,(#64840,#64841,#64842,#64843,#64844,
#64845,#64846,#64847,#64848,#64849,#64850,#64851,#64852,#64853,#64854,#64855,
#64856,#64857,#64858,#64859,#64860,#64861,#64862,#64863,#64864),
 .UNSPECIFIED.,.F.,.F.,(4,3,3,3,3,3,3,3,4),(4.32144212904479E-15,0.172314051943978,
0.344469545399341,0.497068126790716,0.646463497421989,0.7958397759613,0.945404528325424,
0.994136253581434,1.11639350868616),.UNSPECIFIED.);
#922=B_SPLINE_CURVE_WITH_KNOTS('',3,(#64866,#64867,#64868,#64869,#64870,
#64871,#64872,#64873,#64874,#64875,#64876,#64877,#64878,#64879,#64880,#64881,
#64882,#64883,#64884,#64885,#64886,#64887,#64888,#64889,#64890,#64891,#64892,
#64893,#64894,#64895,#64896,#64897,#64898,#64899,#64900,#64901,#64902,#64903,
#64904,#64905,#64906,#64907,#64908,#64909,#64910,#64911,#64912,#64913,#64914,
#64915,#64916,#64917,#64918,#64919,#64920,#64921,#64922,#64923,#64924,#64925,
#64926,#64927,#64928,#64929,#64930,#64931,#64932,#64933,#64934,#64935,#64936,
#64937,#64938,#64939,#64940,#64941,#64942,#64943,#64944,#64945,#64946,#64947,
#64948,#64949,#64950,#64951,#64952,#64953,#64954,#64955,#64956,#64957,#64958,
#64959,#64960,#64961,#64962,#64963,#64964,#64965,#64966,#64967,#64968,#64969,
#64970,#64971,#64972,#64973,#64974,#64975,#64976,#64977,#64978,#64979,#64980,
#64981,#64982,#64983,#64984,#64985,#64986,#64987,#64988,#64989,#64990,#64991,
#64992,#64993,#64994,#64995,#64996,#64997,#64998),.UNSPECIFIED.,.F.,.F.,
(4,3,3,3,3,3,3,3,3,3,3,3,3,3,3,3,3,3,3,3,3,3,3,3,3,3,3,3,3,3,3,3,3,3,3,
3,3,3,3,3,3,3,3,3,4),(1.11639350886518,1.26540107529424,1.4142593470189,
1.56320326233909,1.71217655620612,1.8615074690152,1.98827250716287,2.13573320085301,
2.28291060830462,2.42991002969188,2.57695920191632,2.72402208004863,2.87141215415248,
2.98240876074431,3.13149538526514,3.28032540437999,3.42899933538523,3.5777379135382,
3.726501525518,3.87558312345145,3.97654501432575,4.1254948724311,4.27419103796277,
4.4227344671354,4.57134929638097,4.71999277787197,4.86896212241735,4.97068126790718,
5.11928286943791,5.26762208690304,5.41580101787194,5.56404404366028,5.71231106677202,
5.86090261216133,5.96481752148862,6.11365060296603,6.26222531479554,6.41064301553827,
6.55912704817221,6.70763670357741,6.85646952638757,6.95895377507006,7.11967437914505,
7.27955756183248,7.39957853315717),.UNSPECIFIED.);
#923=B_SPLINE_CURVE_WITH_KNOTS('',3,(#65000,#65001,#65002,#65003,#65004,
#65005,#65006,#65007,#65008,#65009),.UNSPECIFIED.,.F.,.F.,(4,1,1,1,1,1,
1,4),(7.39957881586575,7.9530900286515,8.94722628223293,9.94136253581436,
10.9354987893958,11.9296350429772,12.9237712965587,13.6827641230453),
 .UNSPECIFIED.);
#924=B_SPLINE_CURVE_WITH_KNOTS('',3,(#65011,#65012,#65013,#65014,#65015,
#65016,#65017,#65018,#65019,#65020,#65021),.UNSPECIFIED.,.F.,.F.,(4,1,1,
1,1,1,1,1,4),(13.6827641230453,13.9179075501401,14.9120438037215,15.906180057303,
16.9003163108844,17.8944525644659,18.8885888180473,19.8827250716287,19.9659494302249),
 .UNSPECIFIED.);
#925=B_SPLINE_CURVE_WITH_KNOTS('',3,(#65023,#65024,#65025,#65026,#65027,
#65028,#65029,#65030,#65031,#65032),.UNSPECIFIED.,.F.,.F.,(4,1,1,1,1,1,
1,4),(19.9659494302249,20.8768613252102,21.8709975787916,22.865133832373,
23.8592700859545,24.8534063395359,25.8475425931173,26.2491347374045),
 .UNSPECIFIED.);
#926=B_SPLINE_CURVE_WITH_KNOTS('',3,(#65034,#65035,#65036,#65037,#65038,
#65039,#65040,#65041,#65042,#65043),.UNSPECIFIED.,.F.,.F.,(4,1,1,1,1,1,
1,4),(26.2491347374045,26.8416788466988,27.8358151002802,28.8299513538617,
29.8240876074431,30.8182238610245,31.812360114606,32.5323200445841),
 .UNSPECIFIED.);
#927=B_SPLINE_CURVE_WITH_KNOTS('',3,(#65045,#65046,#65047,#65048,#65049,
#65050,#65051,#65052,#65053,#65054,#65055,#65056,#65057,#65058,#65059,#65060,
#65061,#65062,#65063,#65064,#65065,#65066,#65067,#65068,#65069,#65070,#65071,
#65072,#65073,#65074,#65075,#65076,#65077,#65078,#65079,#65080,#65081,#65082,
#65083,#65084,#65085,#65086,#65087,#65088,#65089,#65090,#65091,#65092,#65093,
#65094,#65095,#65096,#65097,#65098,#65099,#65100,#65101,#65102,#65103,#65104,
#65105,#65106,#65107,#65108,#65109,#65110,#65111,#65112,#65113,#65114,#65115,
#65116,#65117,#65118,#65119,#65120,#65121,#65122,#65123,#65124,#65125,#65126,
#65127,#65128,#65129,#65130,#65131,#65132,#65133,#65134,#65135,#65136,#65137,
#65138,#65139,#65140,#65141,#65142,#65143,#65144,#65145,#65146,#65147,#65148,
#65149,#65150,#65151,#65152,#65153,#65154,#65155,#65156,#65157,#65158,#65159,
#65160,#65161,#65162,#65163,#65164,#65165,#65166,#65167,#65168,#65169,#65170,
#65171,#65172,#65173,#65174,#65175,#65176,#65177),.UNSPECIFIED.,.F.,.F.,
(4,3,3,3,3,3,3,3,3,3,3,3,3,3,3,3,3,3,3,3,3,3,3,3,3,3,3,3,3,3,3,3,3,3,3,
3,3,3,3,3,3,3,3,3,4),(32.5323201655523,32.7174086039218,32.8064963681874,
32.9552946125721,33.1038336449076,33.2522149461395,33.4006619248636,33.5491341052137,
33.6979294074392,33.8006326217688,33.9494658632194,34.0980406789765,34.246458427882,
34.3949424236234,34.5434519944777,34.6922846579409,34.7947688753503,34.9433609925112,
35.0916940432564,35.2398701083223,35.3881153077529,35.536387325413,35.6849883028127,
35.7889051289317,35.9378748258775,36.0865838740458,36.235133264314,36.3837435031379,
36.5323764787389,36.681326045038,36.7830413825131,36.9321232017769,37.0809501019115,
37.2296225918539,37.3783622855042,37.5271284470279,37.6762148396121,37.7771776360946,
37.9230522499658,38.0686696788295,38.2141381094229,38.3596761871594,38.5052593174765,
38.6511351639275,38.6910128210415),.UNSPECIFIED.);
#928=B_SPLINE_CURVE_WITH_KNOTS('',3,(#65181,#65182,#65183,#65184,#65185,
#65186,#65187,#65188,#65189,#65190),.UNSPECIFIED.,.F.,.F.,(4,1,1,1,1,1,
1,4),(-40.7595863968389,-40.2625182700482,-39.7654501432575,-38.771313889676,
-37.7771776360946,-36.7830413825131,-35.7889051289317,-35.5088569560286),
 .UNSPECIFIED.);
#929=B_SPLINE_CURVE_WITH_KNOTS('',3,(#65192,#65193,#65194,#65195,#65196,
#65197,#65198,#65199,#65200,#65201),.UNSPECIFIED.,.F.,.F.,(4,1,1,1,1,1,
1,4),(-35.5088569560286,-34.7947688753503,-33.8006326217688,-32.8064963681874,
-31.812360114606,-30.8182238610245,-29.8240876074431,-29.225671648849),
 .UNSPECIFIED.);
#930=B_SPLINE_CURVE_WITH_KNOTS('',3,(#65203,#65204,#65205,#65206,#65207,
#65208,#65209,#65210,#65211,#65212),.UNSPECIFIED.,.F.,.F.,(4,1,1,1,1,1,
1,4),(-29.225671648849,-28.8299513538617,-27.8358151002802,-26.8416788466988,
-25.8475425931173,-24.8534063395359,-23.8592700859545,-22.9424863416694),
 .UNSPECIFIED.);
#931=B_SPLINE_CURVE_WITH_KNOTS('',3,(#65214,#65215,#65216,#65217,#65218,
#65219,#65220,#65221,#65222,#65223,#65224),.UNSPECIFIED.,.F.,.F.,(4,1,1,
1,1,1,1,1,4),(-22.9424863416694,-22.8651338323731,-21.8709975787916,-20.8768613252102,
-19.8827250716287,-18.8885888180473,-17.8944525644659,-16.9003163108844,
-16.6593010344898),.UNSPECIFIED.);
#932=B_SPLINE_CURVE_WITH_KNOTS('',3,(#65226,#65227,#65228,#65229,#65230,
#65231,#65232,#65233,#65234,#65235),.UNSPECIFIED.,.F.,.F.,(4,1,1,1,1,1,
1,4),(-16.6593010344898,-15.906180057303,-14.9120438037215,-13.9179075501401,
-12.9237712965587,-11.9296350429772,-10.9354987893958,-10.3761157273102),
 .UNSPECIFIED.);
#933=B_SPLINE_CURVE_WITH_KNOTS('',3,(#65236,#65237,#65238,#65239,#65240,
#65241,#65242,#65243,#65244,#65245,#65246,#65247,#65248,#65249,#65250,#65251,
#65252,#65253,#65254,#65255,#65256,#65257,#65258,#65259,#65260,#65261,#65262,
#65263,#65264,#65265,#65266,#65267,#65268,#65269,#65270,#65271,#65272,#65273,
#65274,#65275,#65276,#65277,#65278,#65279,#65280,#65281,#65282,#65283,#65284,
#65285,#65286,#65287,#65288,#65289,#65290,#65291,#65292,#65293,#65294,#65295,
#65296,#65297,#65298,#65299,#65300,#65301,#65302,#65303,#65304,#65305,#65306,
#65307,#65308,#65309,#65310,#65311,#65312,#65313,#65314,#65315,#65316,#65317,
#65318,#65319,#65320,#65321,#65322,#65323,#65324,#65325,#65326,#65327,#65328,
#65329,#65330,#65331,#65332,#65333,#65334,#65335,#65336,#65337,#65338,#65339,
#65340,#65341,#65342,#65343,#65344,#65345,#65346,#65347,#65348,#65349,#65350,
#65351,#65352,#65353,#65354,#65355,#65356,#65357,#65358,#65359,#65360,#65361,
#65362,#65363,#65364,#65365,#65366,#65367,#65368),.UNSPECIFIED.,.F.,.F.,
(4,3,3,3,3,3,3,3,3,3,3,3,3,3,3,3,3,3,3,3,3,3,3,3,3,3,3,3,3,3,3,3,3,3,3,
3,3,3,3,3,3,3,3,3,4),(-10.3761154186762,-10.2158546220139,-10.0546622936771,
-9.94136253581437,-9.79257454522795,-9.64404543825574,-9.49567371048497,
-9.34723566986522,-9.1987720858116,-9.04998470033248,-8.94722628223293,
-8.79847343390106,-8.64997952782992,-8.50164295391919,-8.35323959238031,
-8.20481047459631,-8.05605665252681,-7.95309002865149,-7.804291834983,-7.65575285344285,
-7.50737160293488,-7.3589246742507,-7.21045254363333,-7.06165728984481,
-6.95895377507006,-6.81012048303958,-6.66154561725903,-6.51312781903422,
-6.36464377561713,-6.21613415793645,-6.06730144977603,-5.96481752148862,
-5.81622542190058,-5.66789238697528,-5.51971633593897,-5.37147114763442,
-5.22319913949464,-5.07459816886151,-4.97068126790718,-4.82366356325693,
-4.67690419063574,-4.53020116852648,-4.3835521535988,-4.23663812113851,
-4.09293042032931),.UNSPECIFIED.);
#934=B_SPLINE_CURVE_WITH_KNOTS('',3,(#65371,#65372,#65373,#65374,#65375,
#65376,#65377,#65378,#65379,#65380,#65381,#65382,#65383,#65384,#65385,#65386,
#65387,#65388,#65389,#65390,#65391,#65392,#65393,#65394,#65395,#65396,#65397,
#65398,#65399,#65400,#65401,#65402,#65403,#65404),.UNSPECIFIED.,.F.,.F.,
(4,3,3,3,3,3,3,3,3,3,3,4),(45.5747633669549,45.7279460916964,45.8809709137411,
46.0340726659095,46.1872157257738,46.3406852415556,46.4098017231686,46.5617942570585,
46.7135157473756,46.8650726102834,47.0166960136029,47.1238898038469),
 .UNSPECIFIED.);
#935=B_SPLINE_CURVE_WITH_KNOTS('',3,(#65406,#65407,#65408,#65409,#65410,
#65411,#65412,#65413,#65414,#65415,#65416,#65417,#65418,#65419,#65420,#65421,
#65422,#65423,#65424,#65425,#65426,#65427,#65428,#65429,#65430,#65431,#65432,
#65433,#65434,#65435,#65436,#65437,#65438,#65439,#65440,#65441,#65442,#65443,
#65444,#65445,#65446,#65447,#65448,#65449,#65450,#65451,#65452,#65453,#65454,
#65455,#65456,#65457,#65458,#65459,#65460,#65461,#65462,#65463,#65464,#65465,
#65466,#65467,#65468,#65469,#65470,#65471,#65472),.UNSPECIFIED.,.F.,.F.,
(4,3,3,3,3,3,3,3,3,3,3,3,3,3,3,3,3,3,3,3,3,3,4),(47.1238898040689,47.3128509909798,
47.40393797675,47.5575421867538,47.710870940444,47.8640349431444,48.0172667587525,
48.1705331829181,48.3241211524605,48.3980742303315,48.5517950120318,48.7052464258146,
48.8585386455141,49.0119052759824,49.1653104318385,49.3190408342028,49.3922104839129,
49.5426217757813,49.692761485266,49.8462863076115,49.9963515219788,50.1516061483134,
50.306860774648),.UNSPECIFIED.);
#936=B_SPLINE_CURVE_WITH_KNOTS('',3,(#65476,#65477,#65478,#65479,#65480,
#65481,#65482,#65483,#65484,#65485,#65486,#65487,#65488,#65489,#65490,#65491,
#65492,#65493,#65494,#65495,#65496,#65497,#65498,#65499,#65500,#65501,#65502,
#65503,#65504,#65505,#65506,#65507,#65508,#65509,#65510,#65511,#65512,#65513,
#65514,#65515,#65516,#65517,#65518),.UNSPECIFIED.,.F.,.F.,(4,3,3,3,3,3,
3,3,3,3,3,3,3,3,4),(47.1238898040128,47.2782816278034,47.4323697908821,
47.5927359919967,47.7466225144832,47.9005181633557,48.054632188318,48.0738345953407,
48.2280558285865,48.382092629286,48.5360906232682,48.5709027221314,48.7482748367486,
48.9259950495598,49.0679708489221),.UNSPECIFIED.);
#937=B_SPLINE_CURVE_WITH_KNOTS('',3,(#65519,#65520,#65521,#65522,#65523,
#65524,#65525,#65526,#65527,#65528,#65529,#65530,#65531,#65532,#65533,#65534,
#65535,#65536,#65537,#65538,#65539,#65540,#65541,#65542,#65543,#65544,#65545,
#65546,#65547,#65548,#65549,#65550,#65551,#65552,#65553,#65554,#65555),
 .UNSPECIFIED.,.F.,.F.,(4,3,3,3,3,3,3,3,3,3,3,3,4),(45.5743044775645,45.7276698135094,
45.8810880641648,46.0348251362156,46.0855620881778,46.2375386974501,46.3892415635035,
46.5407859647282,46.6924252089547,46.8441117319342,46.9961635381894,47.0796983417592,
47.1238898038469),.UNSPECIFIED.);
#938=B_SPLINE_CURVE_WITH_KNOTS('',3,(#65558,#65559,#65560,#65561),
 .UNSPECIFIED.,.F.,.F.,(4,4),(-0.968477696161942,-0.935071686684093),
 .UNSPECIFIED.);
#939=B_SPLINE_CURVE_WITH_KNOTS('',3,(#65564,#65565,#65566,#65567,#65568,
#65569),.UNSPECIFIED.,.F.,.F.,(4,2,4),(8.52351753051953E-6,0.0223434875386195,
0.0446411083741544),.UNSPECIFIED.);
#940=B_SPLINE_CURVE_WITH_KNOTS('',3,(#65755,#65756,#65757,#65758),
 .UNSPECIFIED.,.F.,.F.,(4,4),(0.,0.000836946426958433),.UNSPECIFIED.);
#941=B_SPLINE_CURVE_WITH_KNOTS('',3,(#65759,#65760,#65761,#65762,#65763,
#65764,#65765,#65766,#65767,#65768,#65769,#65770,#65771,#65772,#65773,#65774,
#65775,#65776,#65777,#65778,#65779,#65780,#65781,#65782,#65783,#65784,#65785,
#65786,#65787,#65788,#65789,#65790,#65791,#65792,#65793,#65794,#65795,#65796,
#65797,#65798,#65799,#65800,#65801,#65802,#65803,#65804,#65805,#65806,#65807,
#65808,#65809,#65810,#65811,#65812,#65813,#65814,#65815,#65816,#65817,#65818,
#65819,#65820,#65821,#65822,#65823,#65824,#65825),.UNSPECIFIED.,.F.,.F.,
(4,3,3,3,3,3,3,3,3,3,3,3,3,3,3,3,3,3,3,3,3,3,4),(0.,0.0393121242914099,
0.117107898720596,0.167166306519262,0.189098627719502,0.208304762061158,
0.258210465370092,0.32305163930505,0.355694799905693,0.380210492454201,
0.409081485034023,0.483065857864488,0.517575161109925,0.554598739699055,
0.575971627854233,0.64977279486791,0.698159307576866,0.728055674524275,
0.746545820285823,0.819560974564155,0.852041521246935,0.875301939868949,
0.922805662986717),.UNSPECIFIED.);
#942=B_SPLINE_CURVE_WITH_KNOTS('',3,(#65826,#65827,#65828,#65829,#65830,
#65831,#65832,#65833,#65834,#65835,#65836,#65837,#65838,#65839,#65840,#65841,
#65842,#65843,#65844,#65845,#65846,#65847,#65848,#65849,#65850,#65851,#65852,
#65853,#65854,#65855,#65856,#65857,#65858,#65859,#65860,#65861,#65862,#65863,
#65864,#65865,#65866,#65867,#65868,#65869,#65870,#65871,#65872,#65873,#65874,
#65875,#65876,#65877,#65878,#65879,#65880,#65881,#65882,#65883,#65884,#65885,
#65886,#65887,#65888,#65889),.UNSPECIFIED.,.F.,.F.,(4,3,3,3,3,3,3,3,3,3,
3,3,3,3,3,3,3,3,3,3,3,4),(-0.968477696161958,-0.93346935475494,-0.87462218483068,
-0.838968787568558,-0.787473146091247,-0.753349378601184,-0.721529105370558,
-0.646900128137883,-0.59677334563425,-0.567483204022971,-0.543548087950493,
-0.480303919736905,-0.421085426012196,-0.392827821972742,-0.362136007930906,
-0.285930318294375,-0.243429944838067,-0.203365840094899,-0.175996194930052,
-0.0982285541899456,-0.0209966080041514,-2.23186798271618E-15),
 .UNSPECIFIED.);
#943=B_SPLINE_CURVE_WITH_KNOTS('',3,(#65895,#65896,#65897,#65898,#65899,
#65900,#65901,#65902,#65903,#65904,#65905,#65906,#65907,#65908,#65909,#65910,
#65911,#65912,#65913,#65914,#65915,#65916,#65917,#65918,#65919,#65920,#65921,
#65922,#65923,#65924,#65925,#65926,#65927,#65928,#65929,#65930,#65931,#65932,
#65933,#65934,#65935,#65936,#65937,#65938,#65939,#65940,#65941,#65942,#65943,
#65944,#65945,#65946,#65947,#65948,#65949,#65950,#65951,#65952,#65953,#65954,
#65955,#65956,#65957,#65958),.UNSPECIFIED.,.F.,.F.,(4,3,3,3,3,3,3,3,3,3,
3,3,3,3,3,3,3,3,3,3,3,4),(-0.953001334118943,-0.926795214108053,-0.867226959656485,
-0.843238497088046,-0.822042260146921,-0.745112575774413,-0.716203876023601,
-0.693609567103274,-0.617312067174212,-0.566983454838404,-0.537479678376499,
-0.514261574452167,-0.450249178495506,-0.393119621046725,-0.34952529407956,
-0.293393258181454,-0.221730948700384,-0.182710666717766,-0.157793989938048,
-0.085628124075386,-0.0150794994075627,-1.37622244676669E-15),
 .UNSPECIFIED.);
#944=B_SPLINE_CURVE_WITH_KNOTS('',3,(#66144,#66145,#66146,#66147),
 .UNSPECIFIED.,.F.,.F.,(4,4),(0.,0.0112420344023245),.UNSPECIFIED.);
#945=B_SPLINE_CURVE_WITH_KNOTS('',3,(#66148,#66149,#66150,#66151),
 .UNSPECIFIED.,.F.,.F.,(4,4),(0.,0.0131288794431488),.UNSPECIFIED.);
#946=B_SPLINE_CURVE_WITH_KNOTS('',3,(#66152,#66153,#66154,#66155,#66156,
#66157,#66158,#66159,#66160,#66161,#66162,#66163,#66164,#66165,#66166,#66167,
#66168,#66169,#66170,#66171,#66172,#66173,#66174,#66175,#66176,#66177,#66178,
#66179,#66180,#66181,#66182,#66183,#66184,#66185,#66186,#66187,#66188,#66189,
#66190,#66191,#66192,#66193,#66194,#66195,#66196,#66197,#66198,#66199,#66200,
#66201,#66202,#66203,#66204,#66205,#66206,#66207,#66208,#66209,#66210,#66211,
#66212,#66213,#66214,#66215),.UNSPECIFIED.,.F.,.F.,(4,3,3,3,3,3,3,3,3,3,
3,3,3,3,3,3,3,3,3,3,3,4),(0.0447297051812948,0.11579384797572,0.169972513625885,
0.195080510370564,0.269055930443271,0.323648223080396,0.345181704722379,
0.365728274421021,0.407621329269858,0.482026226691156,0.487425100991772,
0.524760575111112,0.54632412226274,0.620775662398705,0.672151363956664,
0.703230969871393,0.723527065514623,0.784142853240842,0.821242619777157,
0.858091484337553,0.935825551512836,0.965990216419499),.UNSPECIFIED.);
#1309=CONICAL_SURFACE('',#16920,0.320138837486628,1.0471975511966);
#1310=CONICAL_SURFACE('',#16925,0.1225,1.0267507402002);
#1311=CONICAL_SURFACE('',#16933,0.465,0.785398163397448);
#1312=CONICAL_SURFACE('',#16941,0.69,0.785398163397449);
#1313=CONICAL_SURFACE('',#16945,0.68,0.785398163397449);
#1520=CYLINDRICAL_SURFACE('',#16903,0.4372);
#1521=CYLINDRICAL_SURFACE('',#16905,0.4372);
#1522=CYLINDRICAL_SURFACE('',#16906,0.4372);
#1523=CYLINDRICAL_SURFACE('',#16907,0.4372);
#1524=CYLINDRICAL_SURFACE('',#16908,0.4372);
#1525=CYLINDRICAL_SURFACE('',#16909,0.4372);
#1526=CYLINDRICAL_SURFACE('',#16910,0.4942);
#1527=CYLINDRICAL_SURFACE('',#16913,0.4372);
#1528=CYLINDRICAL_SURFACE('',#16937,0.44);
#1529=CYLINDRICAL_SURFACE('',#16943,0.7);
#1718=FACE_BOUND('',#4064,.T.);
#1719=FACE_BOUND('',#4070,.T.);
#1720=FACE_BOUND('',#4075,.T.);
#2236=CIRCLE('',#16904,0.4372);
#2237=CIRCLE('',#16911,0.4942);
#2238=CIRCLE('',#16912,0.4942);
#2239=CIRCLE('',#16914,0.4372);
#2240=CIRCLE('',#16916,0.44);
#2241=CIRCLE('',#16918,0.4942);
#2242=CIRCLE('',#16919,0.4942);
#2243=CIRCLE('',#16921,0.308675134594813);
#2244=CIRCLE('',#16926,0.243346949651439);
#2245=CIRCLE('',#16932,0.43);
#2246=CIRCLE('',#16935,0.44);
#2247=CIRCLE('',#16936,0.44);
#2248=CIRCLE('',#16938,0.44);
#2249=CIRCLE('',#16940,0.68);
#2250=CIRCLE('',#16942,0.7);
#2251=CIRCLE('',#16944,0.7);
#2252=CIRCLE('',#16946,0.66);
#3055=FACE_OUTER_BOUND('',#4043,.T.);
#3056=FACE_OUTER_BOUND('',#4044,.T.);
#3057=FACE_OUTER_BOUND('',#4045,.T.);
#3058=FACE_OUTER_BOUND('',#4046,.T.);
#3059=FACE_OUTER_BOUND('',#4047,.T.);
#3060=FACE_OUTER_BOUND('',#4048,.T.);
#3061=FACE_OUTER_BOUND('',#4049,.T.);
#3062=FACE_OUTER_BOUND('',#4050,.T.);
#3063=FACE_OUTER_BOUND('',#4051,.T.);
#3064=FACE_OUTER_BOUND('',#4052,.T.);
#3065=FACE_OUTER_BOUND('',#4053,.T.);
#3066=FACE_OUTER_BOUND('',#4054,.T.);
#3067=FACE_OUTER_BOUND('',#4055,.T.);
#3068=FACE_OUTER_BOUND('',#4056,.T.);
#3069=FACE_OUTER_BOUND('',#4057,.T.);
#3070=FACE_OUTER_BOUND('',#4058,.T.);
#3071=FACE_OUTER_BOUND('',#4059,.T.);
#3072=FACE_OUTER_BOUND('',#4060,.T.);
#3073=FACE_OUTER_BOUND('',#4061,.T.);
#3074=FACE_OUTER_BOUND('',#4062,.T.);
#3075=FACE_OUTER_BOUND('',#4063,.T.);
#3076=FACE_OUTER_BOUND('',#4065,.T.);
#3077=FACE_OUTER_BOUND('',#4066,.T.);
#3078=FACE_OUTER_BOUND('',#4067,.T.);
#3079=FACE_OUTER_BOUND('',#4068,.T.);
#3080=FACE_OUTER_BOUND('',#4069,.T.);
#3081=FACE_OUTER_BOUND('',#4071,.T.);
#3082=FACE_OUTER_BOUND('',#4072,.T.);
#3083=FACE_OUTER_BOUND('',#4073,.T.);
#3084=FACE_OUTER_BOUND('',#4074,.T.);
#4043=EDGE_LOOP('',(#13305,#13306,#13307,#13308));
#4044=EDGE_LOOP('',(#13309,#13310,#13311,#13312,#13313,#13314));
#4045=EDGE_LOOP('',(#13315,#13316,#13317,#13318,#13319,#13320));
#4046=EDGE_LOOP('',(#13321,#13322,#13323,#13324,#13325,#13326));
#4047=EDGE_LOOP('',(#13327,#13328,#13329,#13330,#13331,#13332));
#4048=EDGE_LOOP('',(#13333,#13334,#13335,#13336,#13337,#13338));
#4049=EDGE_LOOP('',(#13339,#13340,#13341,#13342,#13343,#13344,#13345,#13346,
#13347,#13348,#13349,#13350,#13351,#13352,#13353,#13354));
#4050=EDGE_LOOP('',(#13355,#13356,#13357,#13358,#13359,#13360));
#4051=EDGE_LOOP('',(#13361,#13362,#13363,#13364));
#4052=EDGE_LOOP('',(#13365,#13366,#13367,#13368,#13369,#13370,#13371,#13372,
#13373,#13374,#13375,#13376,#13377,#13378,#13379,#13380,#13381,#13382,#13383,
#13384,#13385,#13386,#13387,#13388));
#4053=EDGE_LOOP('',(#13389,#13390,#13391,#13392,#13393));
#4054=EDGE_LOOP('',(#13394,#13395,#13396,#13397,#13398,#13399,#13400,#13401,
#13402,#13403,#13404,#13405,#13406,#13407,#13408,#13409,#13410,#13411,#13412,
#13413,#13414,#13415,#13416,#13417,#13418));
#4055=EDGE_LOOP('',(#13419,#13420,#13421,#13422,#13423,#13424,#13425,#13426,
#13427,#13428));
#4056=EDGE_LOOP('',(#13429,#13430,#13431,#13432));
#4057=EDGE_LOOP('',(#13433,#13434,#13435,#13436));
#4058=EDGE_LOOP('',(#13437,#13438,#13439,#13440));
#4059=EDGE_LOOP('',(#13441,#13442,#13443));
#4060=EDGE_LOOP('',(#13444,#13445,#13446,#13447));
#4061=EDGE_LOOP('',(#13448,#13449,#13450,#13451));
#4062=EDGE_LOOP('',(#13452,#13453,#13454,#13455,#13456));
#4063=EDGE_LOOP('',(#13457,#13458,#13459,#13460,#13461,#13462));
#4064=EDGE_LOOP('',(#13463));
#4065=EDGE_LOOP('',(#13464));
#4066=EDGE_LOOP('',(#13465,#13466,#13467,#13468,#13469,#13470,#13471));
#4067=EDGE_LOOP('',(#13472,#13473,#13474,#13475,#13476));
#4068=EDGE_LOOP('',(#13477,#13478,#13479,#13480,#13481,#13482,#13483,#13484));
#4069=EDGE_LOOP('',(#13485));
#4070=EDGE_LOOP('',(#13486));
#4071=EDGE_LOOP('',(#13487,#13488,#13489,#13490));
#4072=EDGE_LOOP('',(#13491,#13492,#13493,#13494));
#4073=EDGE_LOOP('',(#13495,#13496,#13497,#13498));
#4074=EDGE_LOOP('',(#13499));
#4075=EDGE_LOOP('',(#13500));
#4981=LINE('',#63259,#5841);
#4982=LINE('',#63400,#5842);
#4983=LINE('',#63677,#5843);
#4984=LINE('',#63957,#5844);
#4985=LINE('',#64234,#5845);
#4986=LINE('',#64514,#5846);
#4987=LINE('',#66246,#5847);
#4988=LINE('',#66250,#5848);
#4989=LINE('',#66252,#5849);
#4990=LINE('',#66253,#5850);
#4991=LINE('',#66256,#5851);
#4992=LINE('',#66257,#5852);
#4993=LINE('',#66260,#5853);
#4994=LINE('',#66261,#5854);
#4995=LINE('',#66265,#5855);
#4996=LINE('',#66269,#5856);
#4997=LINE('',#66270,#5857);
#4998=LINE('',#66273,#5858);
#4999=LINE('',#66274,#5859);
#5000=LINE('',#66276,#5860);
#5001=LINE('',#66282,#5861);
#5002=LINE('',#66290,#5862);
#5003=LINE('',#66297,#5863);
#5004=LINE('',#66301,#5864);
#5005=LINE('',#66304,#5865);
#5841=VECTOR('',#20134,0.4372);
#5842=VECTOR('',#20139,0.4372);
#5843=VECTOR('',#20142,0.4372);
#5844=VECTOR('',#20145,0.4372);
#5845=VECTOR('',#20148,0.4372);
#5846=VECTOR('',#20151,0.4372);
#5847=VECTOR('',#20174,0.320138837486628);
#5848=VECTOR('',#20179,1.);
#5849=VECTOR('',#20180,1.);
#5850=VECTOR('',#20181,1.);
#5851=VECTOR('',#20184,1.);
#5852=VECTOR('',#20185,1.);
#5853=VECTOR('',#20188,1.);
#5854=VECTOR('',#20189,1.);
#5855=VECTOR('',#20192,0.1225);
#5856=VECTOR('',#20197,1.);
#5857=VECTOR('',#20198,1.);
#5858=VECTOR('',#20201,1.);
#5859=VECTOR('',#20202,1.);
#5860=VECTOR('',#20205,1.);
#5861=VECTOR('',#20214,0.465);
#5862=VECTOR('',#20225,0.44);
#5863=VECTOR('',#20234,0.69);
#5864=VECTOR('',#20239,0.7);
#5865=VECTOR('',#20242,0.68);
#7128=VERTEX_POINT('',#63257);
#7129=VERTEX_POINT('',#63258);
#7130=VERTEX_POINT('',#63260);
#7131=VERTEX_POINT('',#63340);
#7132=VERTEX_POINT('',#63398);
#7133=VERTEX_POINT('',#63399);
#7134=VERTEX_POINT('',#63401);
#7135=VERTEX_POINT('',#63539);
#7136=VERTEX_POINT('',#63675);
#7137=VERTEX_POINT('',#63676);
#7138=VERTEX_POINT('',#63678);
#7139=VERTEX_POINT('',#63816);
#7140=VERTEX_POINT('',#63955);
#7141=VERTEX_POINT('',#63956);
#7142=VERTEX_POINT('',#63958);
#7143=VERTEX_POINT('',#64093);
#7144=VERTEX_POINT('',#64232);
#7145=VERTEX_POINT('',#64233);
#7146=VERTEX_POINT('',#64235);
#7147=VERTEX_POINT('',#64373);
#7148=VERTEX_POINT('',#64512);
#7149=VERTEX_POINT('',#64513);
#7150=VERTEX_POINT('',#64515);
#7151=VERTEX_POINT('',#64653);
#7152=VERTEX_POINT('',#64789);
#7153=VERTEX_POINT('',#64790);
#7154=VERTEX_POINT('',#64837);
#7155=VERTEX_POINT('',#64839);
#7156=VERTEX_POINT('',#64865);
#7157=VERTEX_POINT('',#64999);
#7158=VERTEX_POINT('',#65010);
#7159=VERTEX_POINT('',#65022);
#7160=VERTEX_POINT('',#65033);
#7161=VERTEX_POINT('',#65044);
#7162=VERTEX_POINT('',#65178);
#7163=VERTEX_POINT('',#65180);
#7164=VERTEX_POINT('',#65191);
#7165=VERTEX_POINT('',#65202);
#7166=VERTEX_POINT('',#65213);
#7167=VERTEX_POINT('',#65225);
#7168=VERTEX_POINT('',#65370);
#7169=VERTEX_POINT('',#65405);
#7170=VERTEX_POINT('',#65473);
#7171=VERTEX_POINT('',#65475);
#7172=VERTEX_POINT('',#65557);
#7173=VERTEX_POINT('',#65562);
#7174=VERTEX_POINT('',#65754);
#7175=VERTEX_POINT('',#65891);
#7176=VERTEX_POINT('',#65893);
#7177=VERTEX_POINT('',#66143);
#7178=VERTEX_POINT('',#66217);
#7179=VERTEX_POINT('',#66218);
#7180=VERTEX_POINT('',#66222);
#7181=VERTEX_POINT('',#66226);
#7182=VERTEX_POINT('',#66230);
#7183=VERTEX_POINT('',#66234);
#7184=VERTEX_POINT('',#66238);
#7185=VERTEX_POINT('',#66245);
#7186=VERTEX_POINT('',#66249);
#7187=VERTEX_POINT('',#66251);
#7188=VERTEX_POINT('',#66255);
#7189=VERTEX_POINT('',#66259);
#7190=VERTEX_POINT('',#66263);
#7191=VERTEX_POINT('',#66264);
#7192=VERTEX_POINT('',#66268);
#7193=VERTEX_POINT('',#66272);
#7194=VERTEX_POINT('',#66279);
#7195=VERTEX_POINT('',#66284);
#7196=VERTEX_POINT('',#66288);
#7197=VERTEX_POINT('',#66292);
#7198=VERTEX_POINT('',#66295);
#7199=VERTEX_POINT('',#66299);
#7200=VERTEX_POINT('',#66303);
#9274=EDGE_CURVE('',#7128,#7129,#4981,.T.);
#9275=EDGE_CURVE('',#7130,#7128,#898,.T.);
#9276=EDGE_CURVE('',#7131,#7130,#2236,.T.);
#9277=EDGE_CURVE('',#7131,#7129,#899,.T.);
#9278=EDGE_CURVE('',#7132,#7133,#4982,.T.);
#9279=EDGE_CURVE('',#7134,#7132,#900,.T.);
#9280=EDGE_CURVE('',#7128,#7134,#901,.T.);
#9281=EDGE_CURVE('',#7129,#7135,#902,.T.);
#9282=EDGE_CURVE('',#7135,#7133,#903,.T.);
#9283=EDGE_CURVE('',#7136,#7137,#4983,.T.);
#9284=EDGE_CURVE('',#7138,#7136,#904,.T.);
#9285=EDGE_CURVE('',#7132,#7138,#905,.T.);
#9286=EDGE_CURVE('',#7133,#7139,#906,.T.);
#9287=EDGE_CURVE('',#7139,#7137,#907,.T.);
#9288=EDGE_CURVE('',#7140,#7141,#4984,.T.);
#9289=EDGE_CURVE('',#7142,#7140,#908,.T.);
#9290=EDGE_CURVE('',#7136,#7142,#909,.T.);
#9291=EDGE_CURVE('',#7137,#7143,#910,.T.);
#9292=EDGE_CURVE('',#7143,#7141,#911,.T.);
#9293=EDGE_CURVE('',#7144,#7145,#4985,.T.);
#9294=EDGE_CURVE('',#7146,#7144,#912,.T.);
#9295=EDGE_CURVE('',#7140,#7146,#913,.T.);
#9296=EDGE_CURVE('',#7141,#7147,#914,.T.);
#9297=EDGE_CURVE('',#7147,#7145,#915,.T.);
#9298=EDGE_CURVE('',#7148,#7149,#4986,.T.);
#9299=EDGE_CURVE('',#7150,#7148,#916,.T.);
#9300=EDGE_CURVE('',#7144,#7150,#917,.T.);
#9301=EDGE_CURVE('',#7145,#7151,#918,.T.);
#9302=EDGE_CURVE('',#7151,#7149,#919,.T.);
#9303=EDGE_CURVE('',#7152,#7153,#920,.T.);
#9304=EDGE_CURVE('',#7153,#7154,#2237,.T.);
#9305=EDGE_CURVE('',#7154,#7155,#921,.T.);
#9306=EDGE_CURVE('',#7155,#7156,#922,.T.);
#9307=EDGE_CURVE('',#7156,#7157,#923,.T.);
#9308=EDGE_CURVE('',#7157,#7158,#924,.T.);
#9309=EDGE_CURVE('',#7158,#7159,#925,.T.);
#9310=EDGE_CURVE('',#7159,#7160,#926,.T.);
#9311=EDGE_CURVE('',#7160,#7161,#927,.T.);
#9312=EDGE_CURVE('',#7162,#7161,#2238,.F.);
#9313=EDGE_CURVE('',#7162,#7163,#928,.T.);
#9314=EDGE_CURVE('',#7163,#7164,#929,.T.);
#9315=EDGE_CURVE('',#7164,#7165,#930,.T.);
#9316=EDGE_CURVE('',#7165,#7166,#931,.T.);
#9317=EDGE_CURVE('',#7166,#7167,#932,.T.);
#9318=EDGE_CURVE('',#7167,#7152,#933,.T.);
#9319=EDGE_CURVE('',#7149,#7168,#934,.T.);
#9320=EDGE_CURVE('',#7168,#7169,#935,.T.);
#9321=EDGE_CURVE('',#7170,#7169,#2239,.T.);
#9322=EDGE_CURVE('',#7171,#7170,#936,.T.);
#9323=EDGE_CURVE('',#7148,#7171,#937,.T.);
#9324=EDGE_CURVE('',#7169,#7172,#938,.T.);
#9325=EDGE_CURVE('',#7173,#7172,#2240,.T.);
#9326=EDGE_CURVE('',#7173,#7170,#939,.T.);
#9327=EDGE_CURVE('',#7174,#7173,#940,.T.);
#9328=EDGE_CURVE('',#7161,#7174,#941,.T.);
#9329=EDGE_CURVE('',#7130,#7154,#942,.T.);
#9330=EDGE_CURVE('',#7154,#7175,#2241,.T.);
#9331=EDGE_CURVE('',#7175,#7176,#2242,.T.);
#9332=EDGE_CURVE('',#7176,#7131,#943,.T.);
#9333=EDGE_CURVE('',#7172,#7177,#944,.T.);
#9334=EDGE_CURVE('',#7176,#7153,#945,.T.);
#9335=EDGE_CURVE('',#7177,#7162,#946,.T.);
#9336=EDGE_CURVE('',#7178,#7179,#266,.T.);
#9337=EDGE_CURVE('',#7180,#7178,#267,.T.);
#9338=EDGE_CURVE('',#7181,#7180,#268,.T.);
#9339=EDGE_CURVE('',#7182,#7181,#269,.T.);
#9340=EDGE_CURVE('',#7183,#7182,#270,.T.);
#9341=EDGE_CURVE('',#7184,#7183,#271,.T.);
#9342=EDGE_CURVE('',#7179,#7184,#272,.T.);
#9343=EDGE_CURVE('',#7179,#7185,#4987,.T.);
#9344=EDGE_CURVE('',#7185,#7185,#2243,.T.);
#9345=EDGE_CURVE('',#7183,#7186,#4988,.T.);
#9346=EDGE_CURVE('',#7186,#7187,#4989,.T.);
#9347=EDGE_CURVE('',#7184,#7187,#4990,.T.);
#9348=EDGE_CURVE('',#7182,#7188,#4991,.T.);
#9349=EDGE_CURVE('',#7188,#7186,#4992,.T.);
#9350=EDGE_CURVE('',#7181,#7189,#4993,.T.);
#9351=EDGE_CURVE('',#7189,#7188,#4994,.T.);
#9352=EDGE_CURVE('',#7190,#7191,#4995,.T.);
#9353=EDGE_CURVE('',#7191,#7191,#2244,.T.);
#9354=EDGE_CURVE('',#7180,#7192,#4996,.T.);
#9355=EDGE_CURVE('',#7192,#7189,#4997,.T.);
#9356=EDGE_CURVE('',#7178,#7193,#4998,.T.);
#9357=EDGE_CURVE('',#7193,#7192,#4999,.T.);
#9358=EDGE_CURVE('',#7187,#7193,#5000,.T.);
#9359=EDGE_CURVE('',#7194,#7194,#2245,.T.);
#9360=EDGE_CURVE('',#7175,#7194,#5001,.T.);
#9361=EDGE_CURVE('',#7195,#7174,#2246,.T.);
#9362=EDGE_CURVE('',#7177,#7195,#2247,.T.);
#9363=EDGE_CURVE('',#7196,#7196,#2248,.T.);
#9364=EDGE_CURVE('',#7196,#7195,#5002,.T.);
#9365=EDGE_CURVE('',#7197,#7197,#2249,.T.);
#9366=EDGE_CURVE('',#7198,#7198,#2250,.T.);
#9367=EDGE_CURVE('',#7198,#7197,#5003,.T.);
#9368=EDGE_CURVE('',#7199,#7199,#2251,.T.);
#9369=EDGE_CURVE('',#7199,#7198,#5004,.T.);
#9370=EDGE_CURVE('',#7199,#7200,#5005,.T.);
#9371=EDGE_CURVE('',#7200,#7200,#2252,.T.);
#13305=ORIENTED_EDGE('',*,*,#9274,.F.);
#13306=ORIENTED_EDGE('',*,*,#9275,.F.);
#13307=ORIENTED_EDGE('',*,*,#9276,.F.);
#13308=ORIENTED_EDGE('',*,*,#9277,.T.);
#13309=ORIENTED_EDGE('',*,*,#9278,.F.);
#13310=ORIENTED_EDGE('',*,*,#9279,.F.);
#13311=ORIENTED_EDGE('',*,*,#9280,.F.);
#13312=ORIENTED_EDGE('',*,*,#9274,.T.);
#13313=ORIENTED_EDGE('',*,*,#9281,.T.);
#13314=ORIENTED_EDGE('',*,*,#9282,.T.);
#13315=ORIENTED_EDGE('',*,*,#9283,.F.);
#13316=ORIENTED_EDGE('',*,*,#9284,.F.);
#13317=ORIENTED_EDGE('',*,*,#9285,.F.);
#13318=ORIENTED_EDGE('',*,*,#9278,.T.);
#13319=ORIENTED_EDGE('',*,*,#9286,.T.);
#13320=ORIENTED_EDGE('',*,*,#9287,.T.);
#13321=ORIENTED_EDGE('',*,*,#9288,.F.);
#13322=ORIENTED_EDGE('',*,*,#9289,.F.);
#13323=ORIENTED_EDGE('',*,*,#9290,.F.);
#13324=ORIENTED_EDGE('',*,*,#9283,.T.);
#13325=ORIENTED_EDGE('',*,*,#9291,.T.);
#13326=ORIENTED_EDGE('',*,*,#9292,.T.);
#13327=ORIENTED_EDGE('',*,*,#9293,.F.);
#13328=ORIENTED_EDGE('',*,*,#9294,.F.);
#13329=ORIENTED_EDGE('',*,*,#9295,.F.);
#13330=ORIENTED_EDGE('',*,*,#9288,.T.);
#13331=ORIENTED_EDGE('',*,*,#9296,.T.);
#13332=ORIENTED_EDGE('',*,*,#9297,.T.);
#13333=ORIENTED_EDGE('',*,*,#9298,.F.);
#13334=ORIENTED_EDGE('',*,*,#9299,.F.);
#13335=ORIENTED_EDGE('',*,*,#9300,.F.);
#13336=ORIENTED_EDGE('',*,*,#9293,.T.);
#13337=ORIENTED_EDGE('',*,*,#9301,.T.);
#13338=ORIENTED_EDGE('',*,*,#9302,.T.);
#13339=ORIENTED_EDGE('',*,*,#9303,.T.);
#13340=ORIENTED_EDGE('',*,*,#9304,.T.);
#13341=ORIENTED_EDGE('',*,*,#9305,.T.);
#13342=ORIENTED_EDGE('',*,*,#9306,.T.);
#13343=ORIENTED_EDGE('',*,*,#9307,.T.);
#13344=ORIENTED_EDGE('',*,*,#9308,.T.);
#13345=ORIENTED_EDGE('',*,*,#9309,.T.);
#13346=ORIENTED_EDGE('',*,*,#9310,.T.);
#13347=ORIENTED_EDGE('',*,*,#9311,.T.);
#13348=ORIENTED_EDGE('',*,*,#9312,.F.);
#13349=ORIENTED_EDGE('',*,*,#9313,.T.);
#13350=ORIENTED_EDGE('',*,*,#9314,.T.);
#13351=ORIENTED_EDGE('',*,*,#9315,.T.);
#13352=ORIENTED_EDGE('',*,*,#9316,.T.);
#13353=ORIENTED_EDGE('',*,*,#9317,.T.);
#13354=ORIENTED_EDGE('',*,*,#9318,.T.);
#13355=ORIENTED_EDGE('',*,*,#9298,.T.);
#13356=ORIENTED_EDGE('',*,*,#9319,.T.);
#13357=ORIENTED_EDGE('',*,*,#9320,.T.);
#13358=ORIENTED_EDGE('',*,*,#9321,.F.);
#13359=ORIENTED_EDGE('',*,*,#9322,.F.);
#13360=ORIENTED_EDGE('',*,*,#9323,.F.);
#13361=ORIENTED_EDGE('',*,*,#9324,.T.);
#13362=ORIENTED_EDGE('',*,*,#9325,.F.);
#13363=ORIENTED_EDGE('',*,*,#9326,.T.);
#13364=ORIENTED_EDGE('',*,*,#9321,.T.);
#13365=ORIENTED_EDGE('',*,*,#9327,.F.);
#13366=ORIENTED_EDGE('',*,*,#9328,.F.);
#13367=ORIENTED_EDGE('',*,*,#9311,.F.);
#13368=ORIENTED_EDGE('',*,*,#9310,.F.);
#13369=ORIENTED_EDGE('',*,*,#9309,.F.);
#13370=ORIENTED_EDGE('',*,*,#9308,.F.);
#13371=ORIENTED_EDGE('',*,*,#9307,.F.);
#13372=ORIENTED_EDGE('',*,*,#9306,.F.);
#13373=ORIENTED_EDGE('',*,*,#9305,.F.);
#13374=ORIENTED_EDGE('',*,*,#9329,.F.);
#13375=ORIENTED_EDGE('',*,*,#9275,.T.);
#13376=ORIENTED_EDGE('',*,*,#9280,.T.);
#13377=ORIENTED_EDGE('',*,*,#9279,.T.);
#13378=ORIENTED_EDGE('',*,*,#9285,.T.);
#13379=ORIENTED_EDGE('',*,*,#9284,.T.);
#13380=ORIENTED_EDGE('',*,*,#9290,.T.);
#13381=ORIENTED_EDGE('',*,*,#9289,.T.);
#13382=ORIENTED_EDGE('',*,*,#9295,.T.);
#13383=ORIENTED_EDGE('',*,*,#9294,.T.);
#13384=ORIENTED_EDGE('',*,*,#9300,.T.);
#13385=ORIENTED_EDGE('',*,*,#9299,.T.);
#13386=ORIENTED_EDGE('',*,*,#9323,.T.);
#13387=ORIENTED_EDGE('',*,*,#9322,.T.);
#13388=ORIENTED_EDGE('',*,*,#9326,.F.);
#13389=ORIENTED_EDGE('',*,*,#9330,.T.);
#13390=ORIENTED_EDGE('',*,*,#9331,.T.);
#13391=ORIENTED_EDGE('',*,*,#9332,.T.);
#13392=ORIENTED_EDGE('',*,*,#9276,.T.);
#13393=ORIENTED_EDGE('',*,*,#9329,.T.);
#13394=ORIENTED_EDGE('',*,*,#9333,.F.);
#13395=ORIENTED_EDGE('',*,*,#9324,.F.);
#13396=ORIENTED_EDGE('',*,*,#9320,.F.);
#13397=ORIENTED_EDGE('',*,*,#9319,.F.);
#13398=ORIENTED_EDGE('',*,*,#9302,.F.);
#13399=ORIENTED_EDGE('',*,*,#9301,.F.);
#13400=ORIENTED_EDGE('',*,*,#9297,.F.);
#13401=ORIENTED_EDGE('',*,*,#9296,.F.);
#13402=ORIENTED_EDGE('',*,*,#9292,.F.);
#13403=ORIENTED_EDGE('',*,*,#9291,.F.);
#13404=ORIENTED_EDGE('',*,*,#9287,.F.);
#13405=ORIENTED_EDGE('',*,*,#9286,.F.);
#13406=ORIENTED_EDGE('',*,*,#9282,.F.);
#13407=ORIENTED_EDGE('',*,*,#9281,.F.);
#13408=ORIENTED_EDGE('',*,*,#9277,.F.);
#13409=ORIENTED_EDGE('',*,*,#9332,.F.);
#13410=ORIENTED_EDGE('',*,*,#9334,.T.);
#13411=ORIENTED_EDGE('',*,*,#9303,.F.);
#13412=ORIENTED_EDGE('',*,*,#9318,.F.);
#13413=ORIENTED_EDGE('',*,*,#9317,.F.);
#13414=ORIENTED_EDGE('',*,*,#9316,.F.);
#13415=ORIENTED_EDGE('',*,*,#9315,.F.);
#13416=ORIENTED_EDGE('',*,*,#9314,.F.);
#13417=ORIENTED_EDGE('',*,*,#9313,.F.);
#13418=ORIENTED_EDGE('',*,*,#9335,.F.);
#13419=ORIENTED_EDGE('',*,*,#9336,.F.);
#13420=ORIENTED_EDGE('',*,*,#9337,.F.);
#13421=ORIENTED_EDGE('',*,*,#9338,.F.);
#13422=ORIENTED_EDGE('',*,*,#9339,.F.);
#13423=ORIENTED_EDGE('',*,*,#9340,.F.);
#13424=ORIENTED_EDGE('',*,*,#9341,.F.);
#13425=ORIENTED_EDGE('',*,*,#9342,.F.);
#13426=ORIENTED_EDGE('',*,*,#9343,.T.);
#13427=ORIENTED_EDGE('',*,*,#9344,.F.);
#13428=ORIENTED_EDGE('',*,*,#9343,.F.);
#13429=ORIENTED_EDGE('',*,*,#9341,.T.);
#13430=ORIENTED_EDGE('',*,*,#9345,.T.);
#13431=ORIENTED_EDGE('',*,*,#9346,.T.);
#13432=ORIENTED_EDGE('',*,*,#9347,.F.);
#13433=ORIENTED_EDGE('',*,*,#9340,.T.);
#13434=ORIENTED_EDGE('',*,*,#9348,.T.);
#13435=ORIENTED_EDGE('',*,*,#9349,.T.);
#13436=ORIENTED_EDGE('',*,*,#9345,.F.);
#13437=ORIENTED_EDGE('',*,*,#9339,.T.);
#13438=ORIENTED_EDGE('',*,*,#9350,.T.);
#13439=ORIENTED_EDGE('',*,*,#9351,.T.);
#13440=ORIENTED_EDGE('',*,*,#9348,.F.);
#13441=ORIENTED_EDGE('',*,*,#9352,.T.);
#13442=ORIENTED_EDGE('',*,*,#9353,.F.);
#13443=ORIENTED_EDGE('',*,*,#9352,.F.);
#13444=ORIENTED_EDGE('',*,*,#9338,.T.);
#13445=ORIENTED_EDGE('',*,*,#9354,.T.);
#13446=ORIENTED_EDGE('',*,*,#9355,.T.);
#13447=ORIENTED_EDGE('',*,*,#9350,.F.);
#13448=ORIENTED_EDGE('',*,*,#9337,.T.);
#13449=ORIENTED_EDGE('',*,*,#9356,.T.);
#13450=ORIENTED_EDGE('',*,*,#9357,.T.);
#13451=ORIENTED_EDGE('',*,*,#9354,.F.);
#13452=ORIENTED_EDGE('',*,*,#9336,.T.);
#13453=ORIENTED_EDGE('',*,*,#9342,.T.);
#13454=ORIENTED_EDGE('',*,*,#9347,.T.);
#13455=ORIENTED_EDGE('',*,*,#9358,.T.);
#13456=ORIENTED_EDGE('',*,*,#9356,.F.);
#13457=ORIENTED_EDGE('',*,*,#9351,.F.);
#13458=ORIENTED_EDGE('',*,*,#9355,.F.);
#13459=ORIENTED_EDGE('',*,*,#9357,.F.);
#13460=ORIENTED_EDGE('',*,*,#9358,.F.);
#13461=ORIENTED_EDGE('',*,*,#9346,.F.);
#13462=ORIENTED_EDGE('',*,*,#9349,.F.);
#13463=ORIENTED_EDGE('',*,*,#9353,.T.);
#13464=ORIENTED_EDGE('',*,*,#9359,.F.);
#13465=ORIENTED_EDGE('',*,*,#9334,.F.);
#13466=ORIENTED_EDGE('',*,*,#9331,.F.);
#13467=ORIENTED_EDGE('',*,*,#9360,.T.);
#13468=ORIENTED_EDGE('',*,*,#9359,.T.);
#13469=ORIENTED_EDGE('',*,*,#9360,.F.);
#13470=ORIENTED_EDGE('',*,*,#9330,.F.);
#13471=ORIENTED_EDGE('',*,*,#9304,.F.);
#13472=ORIENTED_EDGE('',*,*,#9328,.T.);
#13473=ORIENTED_EDGE('',*,*,#9361,.F.);
#13474=ORIENTED_EDGE('',*,*,#9362,.F.);
#13475=ORIENTED_EDGE('',*,*,#9335,.T.);
#13476=ORIENTED_EDGE('',*,*,#9312,.T.);
#13477=ORIENTED_EDGE('',*,*,#9363,.F.);
#13478=ORIENTED_EDGE('',*,*,#9364,.T.);
#13479=ORIENTED_EDGE('',*,*,#9361,.T.);
#13480=ORIENTED_EDGE('',*,*,#9327,.T.);
#13481=ORIENTED_EDGE('',*,*,#9325,.T.);
#13482=ORIENTED_EDGE('',*,*,#9333,.T.);
#13483=ORIENTED_EDGE('',*,*,#9362,.T.);
#13484=ORIENTED_EDGE('',*,*,#9364,.F.);
#13485=ORIENTED_EDGE('',*,*,#9365,.F.);
#13486=ORIENTED_EDGE('',*,*,#9363,.T.);
#13487=ORIENTED_EDGE('',*,*,#9366,.F.);
#13488=ORIENTED_EDGE('',*,*,#9367,.T.);
#13489=ORIENTED_EDGE('',*,*,#9365,.T.);
#13490=ORIENTED_EDGE('',*,*,#9367,.F.);
#13491=ORIENTED_EDGE('',*,*,#9368,.F.);
#13492=ORIENTED_EDGE('',*,*,#9369,.T.);
#13493=ORIENTED_EDGE('',*,*,#9366,.T.);
#13494=ORIENTED_EDGE('',*,*,#9369,.F.);
#13495=ORIENTED_EDGE('',*,*,#9368,.T.);
#13496=ORIENTED_EDGE('',*,*,#9370,.T.);
#13497=ORIENTED_EDGE('',*,*,#9371,.F.);
#13498=ORIENTED_EDGE('',*,*,#9370,.F.);
#13499=ORIENTED_EDGE('',*,*,#9371,.T.);
#13500=ORIENTED_EDGE('',*,*,#9344,.T.);
#14673=PLANE('',#16915);
#14674=PLANE('',#16917);
#14675=PLANE('',#16922);
#14676=PLANE('',#16923);
#14677=PLANE('',#16924);
#14678=PLANE('',#16927);
#14679=PLANE('',#16928);
#14680=PLANE('',#16929);
#14681=PLANE('',#16930);
#14682=PLANE('',#16931);
#14683=PLANE('',#16934);
#14684=PLANE('',#16939);
#14685=PLANE('',#16947);
#15411=ADVANCED_FACE('',(#3055),#1520,.T.);
#15412=ADVANCED_FACE('',(#3056),#1521,.T.);
#15413=ADVANCED_FACE('',(#3057),#1522,.T.);
#15414=ADVANCED_FACE('',(#3058),#1523,.T.);
#15415=ADVANCED_FACE('',(#3059),#1524,.T.);
#15416=ADVANCED_FACE('',(#3060),#1525,.T.);
#15417=ADVANCED_FACE('',(#3061),#1526,.T.);
#15418=ADVANCED_FACE('',(#3062),#1527,.T.);
#15419=ADVANCED_FACE('',(#3063),#14673,.F.);
#15420=ADVANCED_FACE('',(#3064),#254,.F.);
#15421=ADVANCED_FACE('',(#3065),#14674,.T.);
#15422=ADVANCED_FACE('',(#3066),#255,.F.);
#15423=ADVANCED_FACE('',(#3067),#1309,.F.);
#15424=ADVANCED_FACE('',(#3068),#14675,.F.);
#15425=ADVANCED_FACE('',(#3069),#14676,.F.);
#15426=ADVANCED_FACE('',(#3070),#14677,.F.);
#15427=ADVANCED_FACE('',(#3071),#1310,.F.);
#15428=ADVANCED_FACE('',(#3072),#14678,.F.);
#15429=ADVANCED_FACE('',(#3073),#14679,.F.);
#15430=ADVANCED_FACE('',(#3074),#14680,.F.);
#15431=ADVANCED_FACE('',(#3075,#1718),#14681,.F.);
#15432=ADVANCED_FACE('',(#3076),#14682,.T.);
#15433=ADVANCED_FACE('',(#3077),#1311,.T.);
#15434=ADVANCED_FACE('',(#3078),#14683,.T.);
#15435=ADVANCED_FACE('',(#3079),#1528,.T.);
#15436=ADVANCED_FACE('',(#3080,#1719),#14684,.T.);
#15437=ADVANCED_FACE('',(#3081),#1312,.T.);
#15438=ADVANCED_FACE('',(#3082),#1529,.T.);
#15439=ADVANCED_FACE('',(#3083),#1313,.T.);
#15440=ADVANCED_FACE('',(#3084,#1720),#14685,.T.);
#15621=CLOSED_SHELL('',(#15411,#15412,#15413,#15414,#15415,#15416,#15417,
#15418,#15419,#15420,#15421,#15422,#15423,#15424,#15425,#15426,#15427,#15428,
#15429,#15430,#15431,#15432,#15433,#15434,#15435,#15436,#15437,#15438,#15439,
#15440));
#16902=AXIS2_PLACEMENT_3D('',#63255,#20130,#20131);
#16903=AXIS2_PLACEMENT_3D('',#63256,#20132,#20133);
#16904=AXIS2_PLACEMENT_3D('',#63341,#20135,#20136);
#16905=AXIS2_PLACEMENT_3D('',#63397,#20137,#20138);
#16906=AXIS2_PLACEMENT_3D('',#63674,#20140,#20141);
#16907=AXIS2_PLACEMENT_3D('',#63954,#20143,#20144);
#16908=AXIS2_PLACEMENT_3D('',#64231,#20146,#20147);
#16909=AXIS2_PLACEMENT_3D('',#64511,#20149,#20150);
#16910=AXIS2_PLACEMENT_3D('',#64788,#20152,#20153);
#16911=AXIS2_PLACEMENT_3D('',#64838,#20154,#20155);
#16912=AXIS2_PLACEMENT_3D('',#65179,#20156,#20157);
#16913=AXIS2_PLACEMENT_3D('',#65369,#20158,#20159);
#16914=AXIS2_PLACEMENT_3D('',#65474,#20160,#20161);
#16915=AXIS2_PLACEMENT_3D('',#65556,#20162,#20163);
#16916=AXIS2_PLACEMENT_3D('',#65563,#20164,#20165);
#16917=AXIS2_PLACEMENT_3D('',#65890,#20166,#20167);
#16918=AXIS2_PLACEMENT_3D('',#65892,#20168,#20169);
#16919=AXIS2_PLACEMENT_3D('',#65894,#20170,#20171);
#16920=AXIS2_PLACEMENT_3D('',#66216,#20172,#20173);
#16921=AXIS2_PLACEMENT_3D('',#66247,#20175,#20176);
#16922=AXIS2_PLACEMENT_3D('',#66248,#20177,#20178);
#16923=AXIS2_PLACEMENT_3D('',#66254,#20182,#20183);
#16924=AXIS2_PLACEMENT_3D('',#66258,#20186,#20187);
#16925=AXIS2_PLACEMENT_3D('',#66262,#20190,#20191);
#16926=AXIS2_PLACEMENT_3D('',#66266,#20193,#20194);
#16927=AXIS2_PLACEMENT_3D('',#66267,#20195,#20196);
#16928=AXIS2_PLACEMENT_3D('',#66271,#20199,#20200);
#16929=AXIS2_PLACEMENT_3D('',#66275,#20203,#20204);
#16930=AXIS2_PLACEMENT_3D('',#66277,#20206,#20207);
#16931=AXIS2_PLACEMENT_3D('',#66278,#20208,#20209);
#16932=AXIS2_PLACEMENT_3D('',#66280,#20210,#20211);
#16933=AXIS2_PLACEMENT_3D('',#66281,#20212,#20213);
#16934=AXIS2_PLACEMENT_3D('',#66283,#20215,#20216);
#16935=AXIS2_PLACEMENT_3D('',#66285,#20217,#20218);
#16936=AXIS2_PLACEMENT_3D('',#66286,#20219,#20220);
#16937=AXIS2_PLACEMENT_3D('',#66287,#20221,#20222);
#16938=AXIS2_PLACEMENT_3D('',#66289,#20223,#20224);
#16939=AXIS2_PLACEMENT_3D('',#66291,#20226,#20227);
#16940=AXIS2_PLACEMENT_3D('',#66293,#20228,#20229);
#16941=AXIS2_PLACEMENT_3D('',#66294,#20230,#20231);
#16942=AXIS2_PLACEMENT_3D('',#66296,#20232,#20233);
#16943=AXIS2_PLACEMENT_3D('',#66298,#20235,#20236);
#16944=AXIS2_PLACEMENT_3D('',#66300,#20237,#20238);
#16945=AXIS2_PLACEMENT_3D('',#66302,#20240,#20241);
#16946=AXIS2_PLACEMENT_3D('',#66305,#20243,#20244);
#16947=AXIS2_PLACEMENT_3D('',#66306,#20245,#20246);
#20130=DIRECTION('axis',(0.,0.,1.));
#20131=DIRECTION('refdir',(1.,0.,0.));
#20132=DIRECTION('center_axis',(0.,0.,1.));
#20133=DIRECTION('ref_axis',(0.0211112976229345,-0.999777131721203,0.));
#20134=DIRECTION('',(0.,0.,-1.));
#20135=DIRECTION('center_axis',(0.,0.,-1.));
#20136=DIRECTION('ref_axis',(1.,8.30866031508266E-15,0.));
#20137=DIRECTION('center_axis',(0.,0.,1.));
#20138=DIRECTION('ref_axis',(0.0211112976229345,-0.999777131721203,0.));
#20139=DIRECTION('',(0.,0.,-1.));
#20140=DIRECTION('center_axis',(0.,0.,1.));
#20141=DIRECTION('ref_axis',(0.0211112976229345,-0.999777131721203,0.));
#20142=DIRECTION('',(0.,0.,-1.));
#20143=DIRECTION('center_axis',(0.,0.,1.));
#20144=DIRECTION('ref_axis',(0.0211112976229345,-0.999777131721203,0.));
#20145=DIRECTION('',(0.,0.,-1.));
#20146=DIRECTION('center_axis',(0.,0.,1.));
#20147=DIRECTION('ref_axis',(0.0211112976229345,-0.999777131721203,0.));
#20148=DIRECTION('',(0.,0.,-1.));
#20149=DIRECTION('center_axis',(0.,0.,1.));
#20150=DIRECTION('ref_axis',(0.0211112976229345,-0.999777131721203,0.));
#20151=DIRECTION('',(0.,0.,-1.));
#20152=DIRECTION('center_axis',(0.,0.,1.));
#20153=DIRECTION('ref_axis',(1.,0.,0.));
#20154=DIRECTION('center_axis',(0.,0.,1.));
#20155=DIRECTION('ref_axis',(1.,0.,0.));
#20156=DIRECTION('center_axis',(0.,0.,-1.));
#20157=DIRECTION('ref_axis',(1.,0.,0.));
#20158=DIRECTION('center_axis',(0.,0.,1.));
#20159=DIRECTION('ref_axis',(0.0211112976229345,-0.999777131721203,0.));
#20160=DIRECTION('center_axis',(0.,0.,1.));
#20161=DIRECTION('ref_axis',(1.,8.30866031508266E-15,0.));
#20162=DIRECTION('center_axis',(0.,0.,1.));
#20163=DIRECTION('ref_axis',(1.,0.,0.));
#20164=DIRECTION('center_axis',(0.,0.,1.));
#20165=DIRECTION('ref_axis',(1.,0.,0.));
#20166=DIRECTION('center_axis',(0.,0.,1.));
#20167=DIRECTION('ref_axis',(1.,0.,0.));
#20168=DIRECTION('center_axis',(0.,0.,1.));
#20169=DIRECTION('ref_axis',(1.,0.,0.));
#20170=DIRECTION('center_axis',(0.,0.,1.));
#20171=DIRECTION('ref_axis',(1.,0.,0.));
#20172=DIRECTION('center_axis',(0.,0.,1.));
#20173=DIRECTION('ref_axis',(1.,0.,0.));
#20174=DIRECTION('',(-0.86602540378444,-1.06057523872491E-16,0.499999999999998));
#20175=DIRECTION('center_axis',(0.,0.,-1.));
#20176=DIRECTION('ref_axis',(1.,0.,0.));
#20177=DIRECTION('center_axis',(-0.5,-0.866025403784439,0.));
#20178=DIRECTION('ref_axis',(-0.866025403784439,0.5,0.));
#20179=DIRECTION('',(0.,0.,-1.));
#20180=DIRECTION('',(-0.866025403784439,0.5,0.));
#20181=DIRECTION('',(0.,0.,-1.));
#20182=DIRECTION('center_axis',(0.5,-0.866025403784439,0.));
#20183=DIRECTION('ref_axis',(-0.866025403784439,-0.5,0.));
#20184=DIRECTION('',(0.,0.,-1.));
#20185=DIRECTION('',(-0.866025403784439,-0.5,0.));
#20186=DIRECTION('center_axis',(1.,-3.84592537276713E-16,0.));
#20187=DIRECTION('ref_axis',(-3.84592537276713E-16,-1.,0.));
#20188=DIRECTION('',(0.,0.,-1.));
#20189=DIRECTION('',(-3.84592537276713E-16,-1.,0.));
#20190=DIRECTION('center_axis',(0.,0.,1.));
#20191=DIRECTION('ref_axis',(1.,0.,0.));
#20192=DIRECTION('',(-0.855621686410732,-1.04783435954396E-16,0.517601709564076));
#20193=DIRECTION('center_axis',(0.,0.,-1.));
#20194=DIRECTION('ref_axis',(1.,0.,0.));
#20195=DIRECTION('center_axis',(0.5,0.866025403784439,0.));
#20196=DIRECTION('ref_axis',(0.866025403784439,-0.5,0.));
#20197=DIRECTION('',(0.,0.,-1.));
#20198=DIRECTION('',(0.866025403784439,-0.5,0.));
#20199=DIRECTION('center_axis',(-0.5,0.866025403784439,0.));
#20200=DIRECTION('ref_axis',(0.866025403784439,0.5,0.));
#20201=DIRECTION('',(0.,0.,-1.));
#20202=DIRECTION('',(0.866025403784439,0.5,0.));
#20203=DIRECTION('center_axis',(-1.,-1.92296268638356E-16,0.));
#20204=DIRECTION('ref_axis',(-1.92296268638356E-16,1.,0.));
#20205=DIRECTION('',(-1.92296268638356E-16,1.,0.));
#20206=DIRECTION('center_axis',(0.,0.,-1.));
#20207=DIRECTION('ref_axis',(-1.,0.,0.));
#20208=DIRECTION('center_axis',(0.,0.,-1.));
#20209=DIRECTION('ref_axis',(-1.,0.,0.));
#20210=DIRECTION('center_axis',(0.,0.,1.));
#20211=DIRECTION('ref_axis',(1.,0.,0.));
#20212=DIRECTION('center_axis',(0.,0.,1.));
#20213=DIRECTION('ref_axis',(1.,0.,0.));
#20214=DIRECTION('',(0.707106781186547,8.65956056235493E-17,-0.707106781186548));
#20215=DIRECTION('center_axis',(0.,0.,1.));
#20216=DIRECTION('ref_axis',(1.,0.,0.));
#20217=DIRECTION('center_axis',(0.,0.,1.));
#20218=DIRECTION('ref_axis',(1.,0.,0.));
#20219=DIRECTION('center_axis',(0.,0.,1.));
#20220=DIRECTION('ref_axis',(1.,0.,0.));
#20221=DIRECTION('center_axis',(0.,0.,1.));
#20222=DIRECTION('ref_axis',(1.,0.,0.));
#20223=DIRECTION('center_axis',(0.,0.,1.));
#20224=DIRECTION('ref_axis',(1.,0.,0.));
#20225=DIRECTION('',(0.,0.,-1.));
#20226=DIRECTION('center_axis',(0.,0.,-1.));
#20227=DIRECTION('ref_axis',(-1.,0.,0.));
#20228=DIRECTION('center_axis',(0.,0.,1.));
#20229=DIRECTION('ref_axis',(1.,0.,0.));
#20230=DIRECTION('center_axis',(0.,0.,1.));
#20231=DIRECTION('ref_axis',(1.,0.,0.));
#20232=DIRECTION('center_axis',(0.,0.,1.));
#20233=DIRECTION('ref_axis',(1.,0.,0.));
#20234=DIRECTION('',(0.707106781186548,8.65956056235494E-17,-0.707106781186547));
#20235=DIRECTION('center_axis',(0.,0.,1.));
#20236=DIRECTION('ref_axis',(1.,0.,0.));
#20237=DIRECTION('center_axis',(0.,0.,1.));
#20238=DIRECTION('ref_axis',(1.,0.,0.));
#20239=DIRECTION('',(0.,0.,-1.));
#20240=DIRECTION('center_axis',(0.,0.,-1.));
#20241=DIRECTION('ref_axis',(1.,0.,0.));
#20242=DIRECTION('',(0.707106781186548,-8.65956056235494E-17,0.707106781186547));
#20243=DIRECTION('center_axis',(0.,0.,1.));
#20244=DIRECTION('ref_axis',(1.,0.,0.));
#20245=DIRECTION('center_axis',(0.,0.,1.));
#20246=DIRECTION('ref_axis',(1.,0.,0.));
#63255=CARTESIAN_POINT('',(0.,0.,0.));
#63256=CARTESIAN_POINT('Origin',(0.,0.,-0.920658989190502));
#63257=CARTESIAN_POINT('',(-0.00922985932074701,0.43710256198851,-0.675612757771509));
#63258=CARTESIAN_POINT('',(-0.00922985932074692,0.43710256198851,-0.695322262895625));
#63259=CARTESIAN_POINT('',(-0.00922985932074702,0.43710256198851,-0.920658989190502));
#63260=CARTESIAN_POINT('',(-0.253836275241718,-0.35596486536091,-0.73578659827137));
#63261=CARTESIAN_POINT('Ctrl Pts',(-0.253836275241718,-0.35596486536091,
-0.73578659827137));
#63262=CARTESIAN_POINT('Ctrl Pts',(-0.23609314335769,-0.368617379546539,
-0.734988690310258));
#63263=CARTESIAN_POINT('Ctrl Pts',(-0.217340678724491,-0.379983145122343,
-0.734190782349146));
#63264=CARTESIAN_POINT('Ctrl Pts',(-0.197795612701048,-0.389898365726528,
-0.733392874388034));
#63265=CARTESIAN_POINT('Ctrl Pts',(-0.178285302760331,-0.399795954554633,
-0.732596385309573));
#63266=CARTESIAN_POINT('Ctrl Pts',(-0.157985814170068,-0.408247724716953,
-0.731799896231113));
#63267=CARTESIAN_POINT('Ctrl Pts',(-0.13714195136672,-0.415133623277287,
-0.731003407152653));
#63268=CARTESIAN_POINT('Ctrl Pts',(-0.115855204867377,-0.422165831196564,
-0.730189994530307));
#63269=CARTESIAN_POINT('Ctrl Pts',(-0.0940013712333268,-0.427564424236376,
-0.729376581907962));
#63270=CARTESIAN_POINT('Ctrl Pts',(-0.0718621610207865,-0.431253602667181,
-0.728563169285616));
#63271=CARTESIAN_POINT('Ctrl Pts',(-0.0501929304701205,-0.434864465800608,
-0.727767024098989));
#63272=CARTESIAN_POINT('Ctrl Pts',(-0.0282511020507067,-0.436837780034281,
-0.726970878912363));
#63273=CARTESIAN_POINT('Ctrl Pts',(-0.00630957656052663,-0.437154468401762,
-0.726174733725736));
#63274=CARTESIAN_POINT('Ctrl Pts',(0.0163457770492143,-0.43748145965643,
-0.725352687385531));
#63275=CARTESIAN_POINT('Ctrl Pts',(0.0389999615898507,-0.436042033330408,
-0.724530641045326));
#63276=CARTESIAN_POINT('Ctrl Pts',(0.061355526823022,-0.432873352527352,
-0.723708594705121));
#63277=CARTESIAN_POINT('Ctrl Pts',(0.0837110920561935,-0.429704671724297,
-0.722886548364916));
#63278=CARTESIAN_POINT('Ctrl Pts',(0.10576721131509,-0.424806998274031,
-0.722064502024711));
#63279=CARTESIAN_POINT('Ctrl Pts',(0.127242103991421,-0.41827417679297,
-0.721242455684506));
#63280=CARTESIAN_POINT('Ctrl Pts',(0.148546925876914,-0.411793092106706,
-0.720426919554772));
#63281=CARTESIAN_POINT('Ctrl Pts',(0.169414363182626,-0.403662168059158,
-0.719611383425039));
#63282=CARTESIAN_POINT('Ctrl Pts',(0.189574309742103,-0.393961192360117,
-0.718795847295306));
#63283=CARTESIAN_POINT('Ctrl Pts',(0.209698695316446,-0.38427732862373,
-0.717981749724356));
#63284=CARTESIAN_POINT('Ctrl Pts',(0.229117409464745,-0.373029168092783,
-0.717167652153405));
#63285=CARTESIAN_POINT('Ctrl Pts',(0.247578773794493,-0.360345099545443,
-0.716353554582455));
#63286=CARTESIAN_POINT('Ctrl Pts',(0.266020771766867,-0.347674336851346,
-0.715540311016886));
#63287=CARTESIAN_POINT('Ctrl Pts',(0.283506814660605,-0.333571035915543,
-0.714727067451318));
#63288=CARTESIAN_POINT('Ctrl Pts',(0.299812669558214,-0.318207798729662,
-0.713913823885749));
#63289=CARTESIAN_POINT('Ctrl Pts',(0.316126157215975,-0.302837370022371,
-0.713100199641393));
#63290=CARTESIAN_POINT('Ctrl Pts',(0.33125782248679,-0.286206301894547,
-0.712286575397036));
#63291=CARTESIAN_POINT('Ctrl Pts',(0.345018414943263,-0.268525852293663,
-0.71147295115268));
#63292=CARTESIAN_POINT('Ctrl Pts',(0.358782327805654,-0.250841136432466,
-0.710659130582274));
#63293=CARTESIAN_POINT('Ctrl Pts',(0.371174096206649,-0.232107115550857,
-0.709845310011867));
#63294=CARTESIAN_POINT('Ctrl Pts',(0.3820467077514,-0.21256564420507,-0.709031489441461));
#63295=CARTESIAN_POINT('Ctrl Pts',(0.392942211323343,-0.192983028752224,
-0.708215955391037));
#63296=CARTESIAN_POINT('Ctrl Pts',(0.402311867170909,-0.172590213434354,
-0.707400421340613));
#63297=CARTESIAN_POINT('Ctrl Pts',(0.410055556767824,-0.151651839302494,
-0.706584887290189));
#63298=CARTESIAN_POINT('Ctrl Pts',(0.413741612735028,-0.141685011739698,
-0.706196686792816));
#63299=CARTESIAN_POINT('Ctrl Pts',(0.417059976950239,-0.131594818230247,
-0.705808486295443));
#63300=CARTESIAN_POINT('Ctrl Pts',(0.420003875212337,-0.121410810089629,
-0.70542028579807));
#63301=CARTESIAN_POINT('Ctrl Pts',(0.42618277750005,-0.100035753754183,
-0.704605497810254));
#63302=CARTESIAN_POINT('Ctrl Pts',(0.430742949574895,-0.0781284216398137,
-0.703790709822439));
#63303=CARTESIAN_POINT('Ctrl Pts',(0.433604087624001,-0.0559583344619706,
-0.702975921834623));
#63304=CARTESIAN_POINT('Ctrl Pts',(0.436460231986423,-0.0338269418410514,
-0.702162555936848));
#63305=CARTESIAN_POINT('Ctrl Pts',(0.437623085351083,-0.0114343978593403,
-0.701349190039073));
#63306=CARTESIAN_POINT('Ctrl Pts',(0.437063135300412,0.010938727593921,
-0.700535824141298));
#63307=CARTESIAN_POINT('Ctrl Pts',(0.436503760081961,0.0332888852961096,
-0.699723293226793));
#63308=CARTESIAN_POINT('Ctrl Pts',(0.434225084143321,0.0556189534824457,
-0.698910762312289));
#63309=CARTESIAN_POINT('Ctrl Pts',(0.430249624151161,0.0776472853214116,
-0.698098231397785));
#63310=CARTESIAN_POINT('Ctrl Pts',(0.426272118272563,0.0996869535756465,
-0.697285282331424));
#63311=CARTESIAN_POINT('Ctrl Pts',(0.420596193643256,0.121423869876721,
-0.696472333265063));
#63312=CARTESIAN_POINT('Ctrl Pts',(0.413295843054221,0.142584662969411,
-0.695659384198702));
#63313=CARTESIAN_POINT('Ctrl Pts',(0.405993543982359,0.163751103933591,
-0.69484621815409));
#63314=CARTESIAN_POINT('Ctrl Pts',(0.397066218842823,0.1843404517338,-0.694033052109479));
#63315=CARTESIAN_POINT('Ctrl Pts',(0.386636516520684,0.204098123687483,
-0.693219886064868));
#63316=CARTESIAN_POINT('Ctrl Pts',(0.376184292898921,0.223898459222176,
-0.692404964116246));
#63317=CARTESIAN_POINT('Ctrl Pts',(0.364223591037297,0.242862925444445,
-0.691590042167625));
#63318=CARTESIAN_POINT('Ctrl Pts',(0.350921694804399,0.260763885757994,
-0.690775120219003));
#63319=CARTESIAN_POINT('Ctrl Pts',(0.344517650348058,0.269382096549297,
-0.690382785449881));
#63320=CARTESIAN_POINT('Ctrl Pts',(0.337803352917797,0.277754285510053,
-0.689990450680759));
#63321=CARTESIAN_POINT('Ctrl Pts',(0.330800617403977,0.285857991886089,
-0.689598115911637));
#63322=CARTESIAN_POINT('Ctrl Pts',(0.316290891250969,0.302648938810849,
-0.688785195011078));
#63323=CARTESIAN_POINT('Ctrl Pts',(0.300456998910622,0.318381474757695,
-0.68797227411052));
#63324=CARTESIAN_POINT('Ctrl Pts',(0.283479247888115,0.33284133760215,-0.687159353209962));
#63325=CARTESIAN_POINT('Ctrl Pts',(0.266533027410502,0.347274346044395,
-0.686347942040517));
#63326=CARTESIAN_POINT('Ctrl Pts',(0.248447668655544,0.36043887033087,-0.685536530871072));
#63327=CARTESIAN_POINT('Ctrl Pts',(0.229440609456682,0.372157018920974,
-0.684725119701626));
#63328=CARTESIAN_POINT('Ctrl Pts',(0.210445091826676,0.383868051953779,
-0.683914201241642));
#63329=CARTESIAN_POINT('Ctrl Pts',(0.190529570065128,0.394134040634215,
-0.683103282781657));
#63330=CARTESIAN_POINT('Ctrl Pts',(0.169941306080854,0.402819801508731,
-0.682292364321672));
#63331=CARTESIAN_POINT('Ctrl Pts',(0.14936201662218,0.411501776217333,-0.681481799345035));
#63332=CARTESIAN_POINT('Ctrl Pts',(0.128111228261427,0.418604612966437,
-0.680671234368398));
#63333=CARTESIAN_POINT('Ctrl Pts',(0.106456800455306,0.42404102353053,-0.679860669391761));
#63334=CARTESIAN_POINT('Ctrl Pts',(0.0847714872781761,0.42948518796181,
-0.679048948319002));
#63335=CARTESIAN_POINT('Ctrl Pts',(0.0626820859558504,0.433258018369173,
-0.678237227246242));
#63336=CARTESIAN_POINT('Ctrl Pts',(0.0404683503361822,0.435323043981212,
-0.677425506173482));
#63337=CARTESIAN_POINT('Ctrl Pts',(0.0239323278453153,0.43686025998799,
-0.676821256706158));
#63338=CARTESIAN_POINT('Ctrl Pts',(0.00732768865856914,0.437452191233075,
-0.676217007238833));
#63339=CARTESIAN_POINT('Ctrl Pts',(-0.00922985932074701,0.43710256198851,
-0.675612757771509));
#63340=CARTESIAN_POINT('',(0.253835875722688,-0.355965150255044,-0.7358));
#63341=CARTESIAN_POINT('Origin',(0.,0.,-0.7358));
#63342=CARTESIAN_POINT('Ctrl Pts',(0.253835875722687,-0.355965150255045,
-0.7358));
#63343=CARTESIAN_POINT('Ctrl Pts',(0.274914182552133,-0.340934379773804,
-0.734857571584884));
#63344=CARTESIAN_POINT('Ctrl Pts',(0.294627512029226,-0.3240474366386,-0.733915143169768));
#63345=CARTESIAN_POINT('Ctrl Pts',(0.312694699597163,-0.305558283873699,
-0.732972714754652));
#63346=CARTESIAN_POINT('Ctrl Pts',(0.330744485056812,-0.287086939649135,
-0.732031194075799));
#63347=CARTESIAN_POINT('Ctrl Pts',(0.347151135572132,-0.26701667183279,
-0.731089673396946));
#63348=CARTESIAN_POINT('Ctrl Pts',(0.361671991886951,-0.245636337467659,
-0.730148152718094));
#63349=CARTESIAN_POINT('Ctrl Pts',(0.373286559043319,-0.228535188339421,
-0.729395073497657));
#63350=CARTESIAN_POINT('Ctrl Pts',(0.383695334702161,-0.210596615772003,
-0.72864199427722));
#63351=CARTESIAN_POINT('Ctrl Pts',(0.392792712220016,-0.191983658749498,
-0.727888915056783));
#63352=CARTESIAN_POINT('Ctrl Pts',(0.402665549171227,-0.171784135370104,
-0.72707164344855));
#63353=CARTESIAN_POINT('Ctrl Pts',(0.410982336608168,-0.150808835824164,
-0.726254371840317));
#63354=CARTESIAN_POINT('Ctrl Pts',(0.417635754569863,-0.129322142361088,
-0.725437100232084));
#63355=CARTESIAN_POINT('Ctrl Pts',(0.424288360024729,-0.107838072825331,
-0.724619928428007));
#63356=CARTESIAN_POINT('Ctrl Pts',(0.429277804386253,-0.0858434103456964,
-0.72380275662393));
#63357=CARTESIAN_POINT('Ctrl Pts',(0.432546731640961,-0.0636173321251568,
-0.722985584819852));
#63358=CARTESIAN_POINT('Ctrl Pts',(0.435819780852261,-0.0413632279124443,
-0.722167382602296));
#63359=CARTESIAN_POINT('Ctrl Pts',(0.437367913469084,-0.018877827071933,
-0.72134918038474));
#63360=CARTESIAN_POINT('Ctrl Pts',(0.437185553804755,0.00355408841049547,
-0.720530978167183));
#63361=CARTESIAN_POINT('Ctrl Pts',(0.437144458872794,0.00860914290346409,
-0.720346595482644));
#63362=CARTESIAN_POINT('Ctrl Pts',(0.43701569380716,0.0136614873623527,
-0.720162212798104));
#63363=CARTESIAN_POINT('Ctrl Pts',(0.436799559222696,0.0187078877177015,
-0.719977830113565));
#63364=CARTESIAN_POINT('Ctrl Pts',(0.435833468478675,0.041264577041772,
-0.719153665830307));
#63365=CARTESIAN_POINT('Ctrl Pts',(0.433113968332593,0.0637884349248981,
-0.718329501547049));
#63366=CARTESIAN_POINT('Ctrl Pts',(0.428659807839924,0.0859919132397912,
-0.717505337263792));
#63367=CARTESIAN_POINT('Ctrl Pts',(0.424211114992684,0.108168135970398,
-0.716682184672431));
#63368=CARTESIAN_POINT('Ctrl Pts',(0.418032095436736,0.130024080115696,
-0.71585903208107));
#63369=CARTESIAN_POINT('Ctrl Pts',(0.410192983832772,0.151279727704565,
-0.715035879489709));
#63370=CARTESIAN_POINT('Ctrl Pts',(0.402358358148486,0.172523211781469,
-0.714213197946165));
#63371=CARTESIAN_POINT('Ctrl Pts',(0.392865756473906,0.193166431332994,
-0.713390516402621));
#63372=CARTESIAN_POINT('Ctrl Pts',(0.381834617237782,0.212946390152255,
-0.712567834859076));
#63373=CARTESIAN_POINT('Ctrl Pts',(0.370792523466517,0.232745991571373,
-0.711744336346978));
#63374=CARTESIAN_POINT('Ctrl Pts',(0.358209175667509,0.251680014588842,
-0.710920837834879));
#63375=CARTESIAN_POINT('Ctrl Pts',(0.344249629493799,0.26951072816009,-0.71009733932278));
#63376=CARTESIAN_POINT('Ctrl Pts',(0.330282425057853,0.287351223731319,
-0.709273389036141));
#63377=CARTESIAN_POINT('Ctrl Pts',(0.314937976448905,0.304086685582767,
-0.708449438749502));
#63378=CARTESIAN_POINT('Ctrl Pts',(0.298420829956647,0.319513455503811,
-0.707625488462862));
#63379=CARTESIAN_POINT('Ctrl Pts',(0.281864984291512,0.334976369878523,
-0.706799607685711));
#63380=CARTESIAN_POINT('Ctrl Pts',(0.264131494784984,0.349124036809449,
-0.70597372690856));
#63381=CARTESIAN_POINT('Ctrl Pts',(0.245458067100449,0.361793003380817,
-0.705147846131409));
#63382=CARTESIAN_POINT('Ctrl Pts',(0.237980187223299,0.366866362797672,
-0.70481711749665));
#63383=CARTESIAN_POINT('Ctrl Pts',(0.230351882816712,0.371703090974448,
-0.70448638886189));
#63384=CARTESIAN_POINT('Ctrl Pts',(0.222589516841263,0.376294760782519,
-0.704155660227131));
#63385=CARTESIAN_POINT('Ctrl Pts',(0.203657935596137,0.387493352848033,
-0.703349048423612));
#63386=CARTESIAN_POINT('Ctrl Pts',(0.183815030407178,0.3972974216862,-0.702542436620092));
#63387=CARTESIAN_POINT('Ctrl Pts',(0.1632943380843,0.405559858898302,-0.701735824816572));
#63388=CARTESIAN_POINT('Ctrl Pts',(0.142813510323876,0.413806245070843,
-0.700930779979026));
#63389=CARTESIAN_POINT('Ctrl Pts',(0.121658149897246,0.420516609879964,
-0.70012573514148));
#63390=CARTESIAN_POINT('Ctrl Pts',(0.100086214106577,0.425589696475152,
-0.699320690303934));
#63391=CARTESIAN_POINT('Ctrl Pts',(0.0785346546054127,0.430657991164684,
-0.698516405890804));
#63392=CARTESIAN_POINT('Ctrl Pts',(0.0565679968628827,0.434091867394654,
-0.697712121477673));
#63393=CARTESIAN_POINT('Ctrl Pts',(0.0344593539473663,0.435839870738704,
-0.696907837064543));
#63394=CARTESIAN_POINT('Ctrl Pts',(0.0199309555581142,0.436988547709296,
-0.69637931234157));
#63395=CARTESIAN_POINT('Ctrl Pts',(0.00534155190377906,0.437410251961992,
-0.695850787618598));
#63396=CARTESIAN_POINT('Ctrl Pts',(-0.00922985932074692,0.43710256198851,
-0.695322262895625));
#63397=CARTESIAN_POINT('Origin',(0.,0.,-0.920658989190502));
#63398=CARTESIAN_POINT('',(-0.0092298593207472,0.43710256198851,-0.57559571443739));
#63399=CARTESIAN_POINT('',(-0.00922985932074836,0.43710256198851,-0.595330810493319));
#63400=CARTESIAN_POINT('',(-0.00922985932074702,0.43710256198851,-0.920658989190502));
#63401=CARTESIAN_POINT('',(-0.437199981330587,0.000127767500978009,-0.650941010811321));
#63402=CARTESIAN_POINT('Ctrl Pts',(-0.437199981330602,0.000127767450639139,
-0.650941010809498));
#63403=CARTESIAN_POINT('Ctrl Pts',(-0.437206707008506,-0.0228864371799604,
-0.650107475569003));
#63404=CARTESIAN_POINT('Ctrl Pts',(-0.435391893778402,-0.0458841048713647,
-0.649273940328508));
#63405=CARTESIAN_POINT('Ctrl Pts',(-0.431789350475714,-0.0685696493775565,
-0.648440405088013));
#63406=CARTESIAN_POINT('Ctrl Pts',(-0.428183198960036,-0.0912779151307892,
-0.647606035000459));
#63407=CARTESIAN_POINT('Ctrl Pts',(-0.422785904167437,-0.113672790754695,
-0.646771664912904));
#63408=CARTESIAN_POINT('Ctrl Pts',(-0.415682208654229,-0.135470075693277,
-0.64593729482535));
#63409=CARTESIAN_POINT('Ctrl Pts',(-0.408557536979716,-0.157331724787675,
-0.645100460966437));
#63410=CARTESIAN_POINT('Ctrl Pts',(-0.399716654157924,-0.178591646120379,
-0.644263627107525));
#63411=CARTESIAN_POINT('Ctrl Pts',(-0.389292783329051,-0.198984845774547,
-0.643426793248612));
#63412=CARTESIAN_POINT('Ctrl Pts',(-0.383915028511627,-0.209505853707524,
-0.642995064249852));
#63413=CARTESIAN_POINT('Ctrl Pts',(-0.378116695543855,-0.219796585034483,
-0.642563335251093));
#63414=CARTESIAN_POINT('Ctrl Pts',(-0.371920583669806,-0.229823670327299,
-0.642131606252333));
#63415=CARTESIAN_POINT('Ctrl Pts',(-0.360242219712324,-0.248722611124779,
-0.64131788815282));
#63416=CARTESIAN_POINT('Ctrl Pts',(-0.347086172853866,-0.266783349012772,
-0.640504170053308));
#63417=CARTESIAN_POINT('Ctrl Pts',(-0.332597230391415,-0.283765611616278,
-0.639690451953796));
#63418=CARTESIAN_POINT('Ctrl Pts',(-0.318134186922218,-0.300717518415296,
-0.63887818837587));
#63419=CARTESIAN_POINT('Ctrl Pts',(-0.302343394083982,-0.316594201814829,
-0.638065924797943));
#63420=CARTESIAN_POINT('Ctrl Pts',(-0.28541202189861,-0.331185473346503,
-0.637253661220017));
#63421=CARTESIAN_POINT('Ctrl Pts',(-0.268498651128944,-0.345761231454833,
-0.636442261239805));
#63422=CARTESIAN_POINT('Ctrl Pts',(-0.250447629667843,-0.35905380475023,
-0.635630861259594));
#63423=CARTESIAN_POINT('Ctrl Pts',(-0.231481955973139,-0.370890744099728,
-0.634819461279382));
#63424=CARTESIAN_POINT('Ctrl Pts',(-0.212507201857559,-0.382733350761281,
-0.634007672815564));
#63425=CARTESIAN_POINT('Ctrl Pts',(-0.192617517962916,-0.393118536251465,
-0.633195884351746));
#63426=CARTESIAN_POINT('Ctrl Pts',(-0.172064415822184,-0.401917500001892,
-0.632384095887928));
#63427=CARTESIAN_POINT('Ctrl Pts',(-0.151506287174457,-0.410718615644161,
-0.63157210889153));
#63428=CARTESIAN_POINT('Ctrl Pts',(-0.130285087484214,-0.417932484591169,
-0.630760121895132));
#63429=CARTESIAN_POINT('Ctrl Pts',(-0.108671147300701,-0.423478950768925,
-0.629948134898734));
#63430=CARTESIAN_POINT('Ctrl Pts',(-0.0870107368529557,-0.429037341924109,
-0.629134402119293));
#63431=CARTESIAN_POINT('Ctrl Pts',(-0.0649566050649743,-0.432921042028621,
-0.628320669339852));
#63432=CARTESIAN_POINT('Ctrl Pts',(-0.0427891354973138,-0.435101057092938,
-0.62750693656041));
#63433=CARTESIAN_POINT('Ctrl Pts',(-0.0319151525429824,-0.43617043700467,
-0.627107769828907));
#63434=CARTESIAN_POINT('Ctrl Pts',(-0.0210139566724641,-0.436830661251386,
-0.626708603097403));
#63435=CARTESIAN_POINT('Ctrl Pts',(-0.010118573979996,-0.437082891978869,
-0.6263094363659));
#63436=CARTESIAN_POINT('Ctrl Pts',(0.0120971323446054,-0.4375971909187,
-0.625495534630464));
#63437=CARTESIAN_POINT('Ctrl Pts',(0.0344155954638143,-0.436414896660635,
-0.624681632895029));
#63438=CARTESIAN_POINT('Ctrl Pts',(0.0565563354687885,-0.433526493905899,
-0.623867731159593));
#63439=CARTESIAN_POINT('Ctrl Pts',(0.0786576030299037,-0.4306432405868,
-0.623055280445693));
#63440=CARTESIAN_POINT('Ctrl Pts',(0.100581067681182,-0.426059952861661,
-0.622242829731793));
#63441=CARTESIAN_POINT('Ctrl Pts',(0.122048384613809,-0.419819046510708,
-0.621430379017893));
#63442=CARTESIAN_POINT('Ctrl Pts',(0.143492958568617,-0.413584751921958,
-0.620618789033288));
#63443=CARTESIAN_POINT('Ctrl Pts',(0.16448165293897,-0.405696497122655,
-0.619807199048683));
#63444=CARTESIAN_POINT('Ctrl Pts',(0.184748243534716,-0.396247304736369,
-0.618995609064078));
#63445=CARTESIAN_POINT('Ctrl Pts',(0.205024587099967,-0.386793565078811,
-0.618183628514896));
#63446=CARTESIAN_POINT('Ctrl Pts',(0.224577476372314,-0.375777672622639,
-0.617371647965715));
#63447=CARTESIAN_POINT('Ctrl Pts',(0.243161744224629,-0.363340344781083,
-0.616559667416533));
#63448=CARTESIAN_POINT('Ctrl Pts',(0.261750589070784,-0.350899953834034,
-0.615747486890145));
#63449=CARTESIAN_POINT('Ctrl Pts',(0.279369760744317,-0.337037854520489,
-0.614935306363757));
#63450=CARTESIAN_POINT('Ctrl Pts',(0.295804617117614,-0.321937056723673,
-0.614123125837369));
#63451=CARTESIAN_POINT('Ctrl Pts',(0.312274784376428,-0.30680381431462,
-0.613309200311637));
#63452=CARTESIAN_POINT('Ctrl Pts',(0.327555062329663,-0.290427079341062,
-0.612495274785905));
#63453=CARTESIAN_POINT('Ctrl Pts',(0.341468220043877,-0.273026179514101,
-0.611681349260173));
#63454=CARTESIAN_POINT('Ctrl Pts',(0.348272062052594,-0.264516754431455,
-0.611283321666603));
#63455=CARTESIAN_POINT('Ctrl Pts',(0.354749601097303,-0.255762890076055,
-0.610885294073034));
#63456=CARTESIAN_POINT('Ctrl Pts',(0.360883951753957,-0.246792652577924,
-0.610487266479464));
#63457=CARTESIAN_POINT('Ctrl Pts',(0.373427041870483,-0.228450939884396,
-0.609673407563592));
#63458=CARTESIAN_POINT('Ctrl Pts',(0.384604105896927,-0.209098124000313,
-0.608859548647719));
#63459=CARTESIAN_POINT('Ctrl Pts',(0.394254240566668,-0.188964107161121,
-0.608045689731846));
#63460=CARTESIAN_POINT('Ctrl Pts',(0.403887166674859,-0.168865994221708,
-0.607233282126419));
#63461=CARTESIAN_POINT('Ctrl Pts',(0.411998212385938,-0.147990059600682,
-0.606420874520992));
#63462=CARTESIAN_POINT('Ctrl Pts',(0.418471169710053,-0.126592733288683,
-0.605608466915565));
#63463=CARTESIAN_POINT('Ctrl Pts',(0.424937267919239,-0.105218080804583,
-0.604796920183593));
#63464=CARTESIAN_POINT('Ctrl Pts',(0.429768491061065,-0.0833238068245529,
-0.603985373451621));
#63465=CARTESIAN_POINT('Ctrl Pts',(0.432897661814507,-0.061183775590699,
-0.603173826719649));
#63466=CARTESIAN_POINT('Ctrl Pts',(0.436028339652899,-0.0390330811778364,
-0.602361889126978));
#63467=CARTESIAN_POINT('Ctrl Pts',(0.437455208865004,-0.0166370989373022,
-0.601549951534307));
#63468=CARTESIAN_POINT('Ctrl Pts',(0.437162554732755,0.0057219524230085,
-0.600738013941636));
#63469=CARTESIAN_POINT('Ctrl Pts',(0.43686982848041,0.028086513826494,-0.599925876259475));
#63470=CARTESIAN_POINT('Ctrl Pts',(0.434856776168184,0.0504134114387393,
-0.599113738577314));
#63471=CARTESIAN_POINT('Ctrl Pts',(0.431159779498312,0.072422955911557,
-0.598301600895153));
#63472=CARTESIAN_POINT('Ctrl Pts',(0.427454835427866,0.0944798141046644,
-0.597487717367903));
#63473=CARTESIAN_POINT('Ctrl Pts',(0.422058885916212,0.11621725989166,-0.596673833840652));
#63474=CARTESIAN_POINT('Ctrl Pts',(0.415059155108187,0.137367164056328,
-0.595859950313402));
#63475=CARTESIAN_POINT('Ctrl Pts',(0.411633745076104,0.147717146918554,
-0.595461665739945));
#63476=CARTESIAN_POINT('Ctrl Pts',(0.40782501804362,0.157926696114878,-0.595063381166487));
#63477=CARTESIAN_POINT('Ctrl Pts',(0.403647325398977,0.16796629631641,-0.59466509659303));
#63478=CARTESIAN_POINT('Ctrl Pts',(0.395110849896879,0.188480682716078,
-0.593851263026661));
#63479=CARTESIAN_POINT('Ctrl Pts',(0.384982079822358,0.208401318098998,
-0.593037429460293));
#63480=CARTESIAN_POINT('Ctrl Pts',(0.373365985328546,0.227467977965348,
-0.592223595893924));
#63481=CARTESIAN_POINT('Ctrl Pts',(0.361770617011629,0.246500617880724,
-0.591411214421326));
#63482=CARTESIAN_POINT('Ctrl Pts',(0.348693512632148,0.264681673595572,
-0.590598832948729));
#63483=CARTESIAN_POINT('Ctrl Pts',(0.334286251145077,0.281773920538027,
-0.589786451476131));
#63484=CARTESIAN_POINT('Ctrl Pts',(0.319894269219178,0.298848040369167,
-0.588974931571321));
#63485=CARTESIAN_POINT('Ctrl Pts',(0.304175368342171,0.314835081589508,
-0.588163411666511));
#63486=CARTESIAN_POINT('Ctrl Pts',(0.287322477414341,0.329529412909508,
-0.587351891761701));
#63487=CARTESIAN_POINT('Ctrl Pts',(0.270461484632071,0.34423080837856,-0.586539981727021));
#63488=CARTESIAN_POINT('Ctrl Pts',(0.252465939804094,0.357637768087622,
-0.585728071692341));
#63489=CARTESIAN_POINT('Ctrl Pts',(0.233563836147,0.369583244268862,-0.584916161657661));
#63490=CARTESIAN_POINT('Ctrl Pts',(0.214657084771853,0.381531657647269,
-0.584104051987587));
#63491=CARTESIAN_POINT('Ctrl Pts',(0.194843952325113,0.392017516588651,
-0.583291942317512));
#63492=CARTESIAN_POINT('Ctrl Pts',(0.174378718070393,0.400918823060388,
-0.582479832647437));
#63493=CARTESIAN_POINT('Ctrl Pts',(0.153869495105059,0.409839262320423,
-0.581665977399627));
#63494=CARTESIAN_POINT('Ctrl Pts',(0.132706047056115,0.417168108345919,
-0.580852122151817));
#63495=CARTESIAN_POINT('Ctrl Pts',(0.111160684757035,0.422832286095027,
-0.580038266904007));
#63496=CARTESIAN_POINT('Ctrl Pts',(0.100612520042174,0.42560535062012,-0.579639820171537));
#63497=CARTESIAN_POINT('Ctrl Pts',(0.0899729993074902,0.427980190290949,
-0.579241373439067));
#63498=CARTESIAN_POINT('Ctrl Pts',(0.0792747311758675,0.429952738096868,
-0.578842926706597));
#63499=CARTESIAN_POINT('Ctrl Pts',(0.0574208879911633,0.433982152007093,
-0.578029001284114));
#63500=CARTESIAN_POINT('Ctrl Pts',(0.0351965747481254,0.436352639203792,
-0.577215075861632));
#63501=CARTESIAN_POINT('Ctrl Pts',(0.0128772540754298,0.437010316042398,
-0.576401150439149));
#63502=CARTESIAN_POINT('Ctrl Pts',(0.00551507898827925,0.437227255084029,
-0.576132671771896));
#63503=CARTESIAN_POINT('Ctrl Pts',(-0.00185733207176875,0.437258240301254,
-0.575864193104643));
#63504=CARTESIAN_POINT('Ctrl Pts',(-0.0092298593207472,0.43710256198851,
-0.57559571443739));
#63505=CARTESIAN_POINT('Ctrl Pts',(-0.00922985932074701,0.43710256198851,
-0.675612757771509));
#63506=CARTESIAN_POINT('Ctrl Pts',(-0.0260072006138585,0.436748291587515,
-0.675000487189407));
#63507=CARTESIAN_POINT('Ctrl Pts',(-0.0427360189425501,0.435427294772284,
-0.674388216607305));
#63508=CARTESIAN_POINT('Ctrl Pts',(-0.0592984893725335,0.433159934848706,
-0.673775946025203));
#63509=CARTESIAN_POINT('Ctrl Pts',(-0.0813219580013637,0.430144978211756,
-0.672961796830837));
#63510=CARTESIAN_POINT('Ctrl Pts',(-0.103177495193642,0.425437540065905,
-0.672147647636471));
#63511=CARTESIAN_POINT('Ctrl Pts',(-0.12458652359729,0.419072831543566,
-0.671333498442105));
#63512=CARTESIAN_POINT('Ctrl Pts',(-0.14595746363186,0.412719446345326,
-0.670520797684091));
#63513=CARTESIAN_POINT('Ctrl Pts',(-0.166882778259061,0.404714791959317,
-0.669708096926077));
#63514=CARTESIAN_POINT('Ctrl Pts',(-0.187094255225339,0.395145010928489,
-0.668895396168062));
#63515=CARTESIAN_POINT('Ctrl Pts',(-0.20728436950885,0.385585344754514,
-0.668083554400636));
#63516=CARTESIAN_POINT('Ctrl Pts',(-0.226761489326628,0.374464115613459,
-0.66727171263321));
#63517=CARTESIAN_POINT('Ctrl Pts',(-0.245277409181012,0.361915504704414,
-0.666459870865784));
#63518=CARTESIAN_POINT('Ctrl Pts',(-0.263802228239114,0.349360862626204,
-0.665647638907358));
#63519=CARTESIAN_POINT('Ctrl Pts',(-0.281364322202039,0.33537785401944,
-0.664835406948932));
#63520=CARTESIAN_POINT('Ctrl Pts',(-0.297743847746859,0.320144406680634,
-0.664023174990506));
#63521=CARTESIAN_POINT('Ctrl Pts',(-0.314127408365929,0.304907206602414,
-0.663210742939821));
#63522=CARTESIAN_POINT('Ctrl Pts',(-0.329327318663427,0.288419464249492,
-0.662398310889137));
#63523=CARTESIAN_POINT('Ctrl Pts',(-0.343160581830907,0.270896022631329,
-0.661585878838452));
#63524=CARTESIAN_POINT('Ctrl Pts',(-0.357023492965347,0.253335024117745,
-0.660771705553013));
#63525=CARTESIAN_POINT('Ctrl Pts',(-0.369513504192179,0.234734485300197,
-0.659957532267574));
#63526=CARTESIAN_POINT('Ctrl Pts',(-0.380490314154753,0.215339176264835,
-0.659143358982135));
#63527=CARTESIAN_POINT('Ctrl Pts',(-0.385836360686416,0.205893059865574,
-0.658746831367679));
#63528=CARTESIAN_POINT('Ctrl Pts',(-0.390824175469108,0.196258797900248,
-0.658350303753223));
#63529=CARTESIAN_POINT('Ctrl Pts',(-0.395441669118987,0.18646642143933,
-0.657953776138767));
#63530=CARTESIAN_POINT('Ctrl Pts',(-0.405679523518418,0.164754875732289,
-0.657074599622247));
#63531=CARTESIAN_POINT('Ctrl Pts',(-0.414145038150763,0.142156655082225,
-0.656195423105727));
#63532=CARTESIAN_POINT('Ctrl Pts',(-0.420702760698338,0.118966495875085,
-0.655316246589207));
#63533=CARTESIAN_POINT('Ctrl Pts',(-0.427225743179071,0.095899188416417,
-0.65444172758156));
#63534=CARTESIAN_POINT('Ctrl Pts',(-0.431860855423825,0.0722466731816281,
-0.653567208573913));
#63535=CARTESIAN_POINT('Ctrl Pts',(-0.434521538858847,0.0483205160127569,
-0.652692689566266));
#63536=CARTESIAN_POINT('Ctrl Pts',(-0.436298005924746,0.0323456617085848,
-0.652108796647951));
#63537=CARTESIAN_POINT('Ctrl Pts',(-0.437195269979398,0.016249258772824,
-0.651524903729636));
#63538=CARTESIAN_POINT('Ctrl Pts',(-0.437199981330587,0.0001277675009783,
-0.650941010811321));
#63539=CARTESIAN_POINT('',(-0.437199929076795,0.000249028602953033,-0.670658989188628));
#63540=CARTESIAN_POINT('Ctrl Pts',(-0.00922985932074692,0.43710256198851,
-0.695322262895625));
#63541=CARTESIAN_POINT('Ctrl Pts',(-0.0314070055045328,0.436634269287409,
-0.694517867915448));
#63542=CARTESIAN_POINT('Ctrl Pts',(-0.0535419143035678,0.43447398832484,
-0.693713472935271));
#63543=CARTESIAN_POINT('Ctrl Pts',(-0.0753586276524695,0.43065637953981,
-0.692909077955093));
#63544=CARTESIAN_POINT('Ctrl Pts',(-0.0972255992166277,0.426829976295182,
-0.692102829925127));
#63545=CARTESIAN_POINT('Ctrl Pts',(-0.118772195023262,0.421338777062112,
-0.691296581895161));
#63546=CARTESIAN_POINT('Ctrl Pts',(-0.139733376290776,0.414268540382178,
-0.690490333865195));
#63547=CARTESIAN_POINT('Ctrl Pts',(-0.158424889903764,0.407963865876317,
-0.689771386023696));
#63548=CARTESIAN_POINT('Ctrl Pts',(-0.176650775880943,0.400404465031996,
-0.689052438182196));
#63549=CARTESIAN_POINT('Ctrl Pts',(-0.194238339255865,0.391682661810711,
-0.688333490340697));
#63550=CARTESIAN_POINT('Ctrl Pts',(-0.214188832527874,0.381789064114617,
-0.687517950190592));
#63551=CARTESIAN_POINT('Ctrl Pts',(-0.233436790932398,0.370339900816165,
-0.686702410040488));
#63552=CARTESIAN_POINT('Ctrl Pts',(-0.251728887762749,0.357458259193615,
-0.685886869890383));
#63553=CARTESIAN_POINT('Ctrl Pts',(-0.269988720408491,0.344599338621977,
-0.685072768216042));
#63554=CARTESIAN_POINT('Ctrl Pts',(-0.28729543149376,0.330313317168977,
-0.684258666541701));
#63555=CARTESIAN_POINT('Ctrl Pts',(-0.303421857626618,0.31476819457247,
-0.68344456486736));
#63556=CARTESIAN_POINT('Ctrl Pts',(-0.319531368230129,0.299239377757251,
-0.682631317130566));
#63557=CARTESIAN_POINT('Ctrl Pts',(-0.334462523180116,0.282454554403131,
-0.681818069393772));
#63558=CARTESIAN_POINT('Ctrl Pts',(-0.34802249643644,0.264620826795905,
-0.681004821656977));
#63559=CARTESIAN_POINT('Ctrl Pts',(-0.361588817911958,0.246778750174284,
-0.680191193191195));
#63560=CARTESIAN_POINT('Ctrl Pts',(-0.373782229810875,0.227887344095649,
-0.679377564725412));
#63561=CARTESIAN_POINT('Ctrl Pts',(-0.384450764797267,0.208186093307877,
-0.67856393625963));
#63562=CARTESIAN_POINT('Ctrl Pts',(-0.395121874506069,0.188480087860543,
-0.677750111434418));
#63563=CARTESIAN_POINT('Ctrl Pts',(-0.404267062659073,0.167964489125426,
-0.676936286609206));
#63564=CARTESIAN_POINT('Ctrl Pts',(-0.411781053241527,0.146902022420722,
-0.676122461783995));
#63565=CARTESIAN_POINT('Ctrl Pts',(-0.419310864121166,0.125795209841608,
-0.675306923495018));
#63566=CARTESIAN_POINT('Ctrl Pts',(-0.425202425782493,0.104139916643362,
-0.674491385206042));
#63567=CARTESIAN_POINT('Ctrl Pts',(-0.429400462770177,0.0822136398218577,
-0.673675846917065));
#63568=CARTESIAN_POINT('Ctrl Pts',(-0.431398621626343,0.0717772896081326,
-0.673287671429464));
#63569=CARTESIAN_POINT('Ctrl Pts',(-0.433013865462819,0.0612796736223055,
-0.672899495941863));
#63570=CARTESIAN_POINT('Ctrl Pts',(-0.434244367921488,0.0507510485454944,
-0.672511320454263));
#63571=CARTESIAN_POINT('Ctrl Pts',(-0.436201642613934,0.0340038967914236,
-0.671893876699676));
#63572=CARTESIAN_POINT('Ctrl Pts',(-0.437190307036958,0.017141683576328,
-0.671276432945089));
#63573=CARTESIAN_POINT('Ctrl Pts',(-0.437199929076766,0.000249028654235785,
-0.670658989190502));
#63574=CARTESIAN_POINT('Ctrl Pts',(-0.437199929076795,0.000249028602953033,
-0.670658989188628));
#63575=CARTESIAN_POINT('Ctrl Pts',(-0.437212452159017,-0.0217367617606223,
-0.669855386142677));
#63576=CARTESIAN_POINT('Ctrl Pts',(-0.4355622610073,-0.0437851949110618,
-0.669051783096727));
#63577=CARTESIAN_POINT('Ctrl Pts',(-0.43224731193602,-0.0656208909120047,
-0.668248180050776));
#63578=CARTESIAN_POINT('Ctrl Pts',(-0.428937309510904,-0.0874240031659445,
-0.66744577616048));
#63579=CARTESIAN_POINT('Ctrl Pts',(-0.423967539716265,-0.109014281124924,
-0.666643372270185));
#63580=CARTESIAN_POINT('Ctrl Pts',(-0.417387828497506,-0.130120100761322,
-0.665840968379889));
#63581=CARTESIAN_POINT('Ctrl Pts',(-0.410807504084803,-0.151227887347385,
-0.665038489709837));
#63582=CARTESIAN_POINT('Ctrl Pts',(-0.402617116897674,-0.171850412733853,
-0.664236011039784));
#63583=CARTESIAN_POINT('Ctrl Pts',(-0.392916898071436,-0.191729369711374,
-0.663433532369732));
#63584=CARTESIAN_POINT('Ctrl Pts',(-0.383217301367585,-0.211607051754341,
-0.662631105166554));
#63585=CARTESIAN_POINT('Ctrl Pts',(-0.372008404123178,-0.230740607532142,
-0.661828677963376));
#63586=CARTESIAN_POINT('Ctrl Pts',(-0.359436913400565,-0.248895450511001,
-0.661026250760198));
#63587=CARTESIAN_POINT('Ctrl Pts',(-0.346837793311001,-0.26709019383499,
-0.660222059998812));
#63588=CARTESIAN_POINT('Ctrl Pts',(-0.33287054764678,-0.284301343360384,
-0.659417869237426));
#63589=CARTESIAN_POINT('Ctrl Pts',(-0.317723540675403,-0.300325809248366,
-0.65861367847604));
#63590=CARTESIAN_POINT('Ctrl Pts',(-0.305640653943371,-0.313108651867483,
-0.657972169173303));
#63591=CARTESIAN_POINT('Ctrl Pts',(-0.292807951576093,-0.32513693237376,
-0.657330659870565));
#63592=CARTESIAN_POINT('Ctrl Pts',(-0.279336207285159,-0.336325918269085,
-0.656689150567827));
#63593=CARTESIAN_POINT('Ctrl Pts',(-0.262265604125063,-0.350503944058331,
-0.655876267655708));
#63594=CARTESIAN_POINT('Ctrl Pts',(-0.244062841964013,-0.363420492111987,
-0.655063384743588));
#63595=CARTESIAN_POINT('Ctrl Pts',(-0.224940951780152,-0.374893862596121,
-0.654250501831469));
#63596=CARTESIAN_POINT('Ctrl Pts',(-0.205853665365587,-0.386346470390926,
-0.65343908994614));
#63597=CARTESIAN_POINT('Ctrl Pts',(-0.185851131125435,-0.396360670469547,
-0.652627678060812));
#63598=CARTESIAN_POINT('Ctrl Pts',(-0.165177059889714,-0.404796713037779,
-0.651816266175484));
#63599=CARTESIAN_POINT('Ctrl Pts',(-0.144525341083946,-0.413223634710158,
-0.651005731573934));
#63600=CARTESIAN_POINT('Ctrl Pts',(-0.123204176561203,-0.420075489728682,
-0.650195196972384));
#63601=CARTESIAN_POINT('Ctrl Pts',(-0.101479296768336,-0.425259676347763,
-0.649384662370834));
#63602=CARTESIAN_POINT('Ctrl Pts',(-0.0797442867957068,-0.43044628032164,
-0.648573749821912));
#63603=CARTESIAN_POINT('Ctrl Pts',(-0.0576058788370304,-0.43396347684704,
-0.64776283727299));
#63604=CARTESIAN_POINT('Ctrl Pts',(-0.0353429899867632,-0.435769105213754,
-0.646951924724069));
#63605=CARTESIAN_POINT('Ctrl Pts',(-0.0130748491733914,-0.437575159540172,
-0.6461408208755));
#63606=CARTESIAN_POINT('Ctrl Pts',(0.00931711353290146,-0.437668815182892,
-0.64532971702693));
#63607=CARTESIAN_POINT('Ctrl Pts',(0.0315515946571501,-0.43606001522106,
-0.644518613178361));
#63608=CARTESIAN_POINT('Ctrl Pts',(0.0538340014276071,-0.434447747547192,
-0.643705761023822));
#63609=CARTESIAN_POINT('Ctrl Pts',(0.0759575371609294,-0.431125798174385,
-0.642892908869284));
#63610=CARTESIAN_POINT('Ctrl Pts',(0.0976476401346384,-0.426155814668926,
-0.642080056714745));
#63611=CARTESIAN_POINT('Ctrl Pts',(0.10843752524531,-0.423683463519149,
-0.641675698036961));
#63612=CARTESIAN_POINT('Ctrl Pts',(0.119120351997259,-0.420804075188136,
-0.641271339359178));
#63613=CARTESIAN_POINT('Ctrl Pts',(0.129663922009771,-0.417529768195088,
-0.640866980681394));
#63614=CARTESIAN_POINT('Ctrl Pts',(0.150892702491631,-0.410937167747313,
-0.640052831242787));
#63615=CARTESIAN_POINT('Ctrl Pts',(0.171677745929381,-0.402702679274393,
-0.63923868180418));
#63616=CARTESIAN_POINT('Ctrl Pts',(0.191750046405751,-0.392906807911739,
-0.638424532365573));
#63617=CARTESIAN_POINT('Ctrl Pts',(0.211786636880584,-0.383128364077228,
-0.63761183135475));
#63618=CARTESIAN_POINT('Ctrl Pts',(0.231112341796989,-0.37179431180374,
-0.636799130343927));
#63619=CARTESIAN_POINT('Ctrl Pts',(0.249476747912302,-0.359033692362015,
-0.635986429333104));
#63620=CARTESIAN_POINT('Ctrl Pts',(0.267821743800063,-0.346286560235126,
-0.635174587305221));
#63621=CARTESIAN_POINT('Ctrl Pts',(0.285206858144772,-0.332116237615206,
-0.634362745277338));
#63622=CARTESIAN_POINT('Ctrl Pts',(0.301409305687097,-0.31669586426921,
-0.633550903249455));
#63623=CARTESIAN_POINT('Ctrl Pts',(0.317619540685347,-0.301268079359162,
-0.632738671022252));
#63624=CARTESIAN_POINT('Ctrl Pts',(0.332645442649692,-0.284589522910896,
-0.631926438795049));
#63625=CARTESIAN_POINT('Ctrl Pts',(0.346299390938616,-0.266871826605102,
-0.631114206567846));
#63626=CARTESIAN_POINT('Ctrl Pts',(0.359956702944012,-0.249149765458776,
-0.630301774243289));
#63627=CARTESIAN_POINT('Ctrl Pts',(0.3722409770448,-0.230388640070999,-0.629489341918732));
#63628=CARTESIAN_POINT('Ctrl Pts',(0.383007003794254,-0.21083044145604,
-0.628676909594176));
#63629=CARTESIAN_POINT('Ctrl Pts',(0.393796104733718,-0.191230324907786,
-0.627862736031345));
#63630=CARTESIAN_POINT('Ctrl Pts',(0.40306015939866,-0.170830373667132,
-0.627048562468515));
#63631=CARTESIAN_POINT('Ctrl Pts',(0.410700990773741,-0.149895083900265,
-0.626234388905685));
#63632=CARTESIAN_POINT('Ctrl Pts',(0.414422296306332,-0.139698993211769,
-0.625837862868776));
#63633=CARTESIAN_POINT('Ctrl Pts',(0.417759328118468,-0.12937617521928,
-0.625441336831868));
#63634=CARTESIAN_POINT('Ctrl Pts',(0.420705095541896,-0.118958238828105,
-0.625044810794959));
#63635=CARTESIAN_POINT('Ctrl Pts',(0.426751840268641,-0.0975734541923914,
-0.624230866115));
#63636=CARTESIAN_POINT('Ctrl Pts',(0.431181153288528,-0.0756655031661115,
-0.623416921435041));
#63637=CARTESIAN_POINT('Ctrl Pts',(0.433913816065184,-0.053503646864019,
-0.622602976755082));
#63638=CARTESIAN_POINT('Ctrl Pts',(0.436641616652187,-0.0313812228509463,
-0.621790480315805));
#63639=CARTESIAN_POINT('Ctrl Pts',(0.437678617813652,-0.00900648565784756,
-0.620977983876527));
#63640=CARTESIAN_POINT('Ctrl Pts',(0.436996422614475,0.0133404131176973,
-0.620165487437249));
#63641=CARTESIAN_POINT('Ctrl Pts',(0.436314947907121,0.0356637104990086,
-0.6193538491058));
#63642=CARTESIAN_POINT('Ctrl Pts',(0.43391787560429,0.0579585155943608,
-0.61854221077435));
#63643=CARTESIAN_POINT('Ctrl Pts',(0.429828839422716,0.0799437852526436,
-0.617730572442901));
#63644=CARTESIAN_POINT('Ctrl Pts',(0.425737818513836,0.101939726072318,
-0.61691854016024));
#63645=CARTESIAN_POINT('Ctrl Pts',(0.419953305726717,0.123625124627191,
-0.616106507877578));
#63646=CARTESIAN_POINT('Ctrl Pts',(0.412550375838212,0.144727424477014,
-0.615294475594917));
#63647=CARTESIAN_POINT('Ctrl Pts',(0.405145604587074,0.165834973192759,
-0.614482241331969));
#63648=CARTESIAN_POINT('Ctrl Pts',(0.396121881367468,0.186358470157252,
-0.613670007069021));
#63649=CARTESIAN_POINT('Ctrl Pts',(0.385602853630614,0.20604436238812,-0.612857772806072));
#63650=CARTESIAN_POINT('Ctrl Pts',(0.375061197452133,0.225772602740353,
-0.612043791271792));
#63651=CARTESIAN_POINT('Ctrl Pts',(0.363018194278841,0.244659033216597,
-0.611229809737512));
#63652=CARTESIAN_POINT('Ctrl Pts',(0.349641998044345,0.262477262260102,
-0.610415828203231));
#63653=CARTESIAN_POINT('Ctrl Pts',(0.343106097360962,0.271183636878155,
-0.610018099104996));
#63654=CARTESIAN_POINT('Ctrl Pts',(0.336252519568758,0.279635469956066,
-0.609620370006761));
#63655=CARTESIAN_POINT('Ctrl Pts',(0.329104171259901,0.287809458599494,
-0.609222640908525));
#63656=CARTESIAN_POINT('Ctrl Pts',(0.314478583628286,0.304533515967566,
-0.608408883446165));
#63657=CARTESIAN_POINT('Ctrl Pts',(0.298532990971369,0.320187864219064,
-0.607595125983804));
#63658=CARTESIAN_POINT('Ctrl Pts',(0.281449718780217,0.334559256034767,
-0.606781368521444));
#63659=CARTESIAN_POINT('Ctrl Pts',(0.264397829962196,0.348904246424167,
-0.605969105998331));
#63660=CARTESIAN_POINT('Ctrl Pts',(0.246212916914089,0.361970461363107,
-0.605156843475219));
#63661=CARTESIAN_POINT('Ctrl Pts',(0.227114142122697,0.37358132507912,-0.604344580952106));
#63662=CARTESIAN_POINT('Ctrl Pts',(0.208026932940381,0.385185157626264,
-0.60353281030928));
#63663=CARTESIAN_POINT('Ctrl Pts',(0.188027547854929,0.395334982137295,
-0.602721039666453));
#63664=CARTESIAN_POINT('Ctrl Pts',(0.167364636428823,0.403897163239664,
-0.601909269023626));
#63665=CARTESIAN_POINT('Ctrl Pts',(0.146710493450358,0.412455710921982,
-0.601097842861218));
#63666=CARTESIAN_POINT('Ctrl Pts',(0.125394044635463,0.419427680505348,
-0.60028641669881));
#63667=CARTESIAN_POINT('Ctrl Pts',(0.103684190323387,0.424727475773564,
-0.599474990536402));
#63668=CARTESIAN_POINT('Ctrl Pts',(0.0819443642684749,0.430034587723808,
-0.598662444152001));
#63669=CARTESIAN_POINT('Ctrl Pts',(0.0598107485201382,0.433664759998317,
-0.5978498977676));
#63670=CARTESIAN_POINT('Ctrl Pts',(0.03756375015824,0.435583292464311,-0.597037351383199));
#63671=CARTESIAN_POINT('Ctrl Pts',(0.0219890854947838,0.436926417470108,
-0.596468504419906));
#63672=CARTESIAN_POINT('Ctrl Pts',(0.00635908031257408,0.437431738095647,
-0.595899657456613));
#63673=CARTESIAN_POINT('Ctrl Pts',(-0.00922985932074836,0.43710256198851,
-0.595330810493319));
#63674=CARTESIAN_POINT('Origin',(0.,0.,-0.920658989190502));
#63675=CARTESIAN_POINT('',(-0.00922985932074692,0.43710256198851,-0.475606184023132));
#63676=CARTESIAN_POINT('',(-0.00922985932074758,0.43710256198851,-0.495313704306577));
#63677=CARTESIAN_POINT('',(-0.00922985932074702,0.43710256198851,-0.920658989190502));
#63678=CARTESIAN_POINT('',(-0.437199823825855,-0.000392487759930489,-0.550941010807406));
#63679=CARTESIAN_POINT('Ctrl Pts',(-0.437199823825855,-0.000392487759930985,
-0.550941010807406));
#63680=CARTESIAN_POINT('Ctrl Pts',(-0.437173299123608,-0.0299388745087773,
-0.549865238956156));
#63681=CARTESIAN_POINT('Ctrl Pts',(-0.434147816830185,-0.0593528249596906,
-0.548789467104907));
#63682=CARTESIAN_POINT('Ctrl Pts',(-0.428225193397315,-0.0881307196148554,
-0.547713695253658));
#63683=CARTESIAN_POINT('Ctrl Pts',(-0.42727988992287,-0.0927239280322208,
-0.547541992480348));
#63684=CARTESIAN_POINT('Ctrl Pts',(-0.426260877065074,-0.0973009825016195,
-0.547370289707038));
#63685=CARTESIAN_POINT('Ctrl Pts',(-0.425168676443051,-0.101859886960786,
-0.547198586933727));
#63686=CARTESIAN_POINT('Ctrl Pts',(-0.419991785780037,-0.123468508538497,
-0.546384737842233));
#63687=CARTESIAN_POINT('Ctrl Pts',(-0.413148549881292,-0.144743242971641,
-0.545570888750738));
#63688=CARTESIAN_POINT('Ctrl Pts',(-0.404701375565575,-0.165410509385986,
-0.544757039659243));
#63689=CARTESIAN_POINT('Ctrl Pts',(-0.396269269375605,-0.186040909392995,
-0.543944642317172));
#63690=CARTESIAN_POINT('Ctrl Pts',(-0.386239120277342,-0.20606531629854,
-0.543132244975101));
#63691=CARTESIAN_POINT('Ctrl Pts',(-0.374722999789755,-0.225225472423896,
-0.54231984763303));
#63692=CARTESIAN_POINT('Ctrl Pts',(-0.363219088317679,-0.244365315576356,
-0.541508311568137));
#63693=CARTESIAN_POINT('Ctrl Pts',(-0.350232675903339,-0.262642102451221,
-0.540696775503244));
#63694=CARTESIAN_POINT('Ctrl Pts',(-0.335921668328666,-0.279822216321874,
-0.539885239438351));
#63695=CARTESIAN_POINT('Ctrl Pts',(-0.321603776659083,-0.29701059442786,
-0.539073312996242));
#63696=CARTESIAN_POINT('Ctrl Pts',(-0.305960460555495,-0.31310068390885,
-0.538261386554133));
#63697=CARTESIAN_POINT('Ctrl Pts',(-0.289190361932185,-0.327891406666189,
-0.537449460112023));
#63698=CARTESIAN_POINT('Ctrl Pts',(-0.272416136530548,-0.342685769117932,
-0.536637333871421));
#63699=CARTESIAN_POINT('Ctrl Pts',(-0.254515133900513,-0.356179678793403,
-0.535825207630818));
#63700=CARTESIAN_POINT('Ctrl Pts',(-0.235719089868977,-0.36821237169783,
-0.535013081390215));
#63701=CARTESIAN_POINT('Ctrl Pts',(-0.21688264590535,-0.380270927489969,
-0.534199209577782));
#63702=CARTESIAN_POINT('Ctrl Pts',(-0.197147948073415,-0.390861651227168,
-0.53338533776535));
#63703=CARTESIAN_POINT('Ctrl Pts',(-0.176772290129475,-0.399869225425489,
-0.532571465952917));
#63704=CARTESIAN_POINT('Ctrl Pts',(-0.16679942243077,-0.404277983464777,
-0.532173116317709));
#63705=CARTESIAN_POINT('Ctrl Pts',(-0.15667331020594,-0.408308216793835,
-0.531774766682501));
#63706=CARTESIAN_POINT('Ctrl Pts',(-0.146425481105729,-0.411950747642186,
-0.531376417047293));
#63707=CARTESIAN_POINT('Ctrl Pts',(-0.125488539703116,-0.419392660869208,
-0.53056256438752));
#63708=CARTESIAN_POINT('Ctrl Pts',(-0.103922955068954,-0.425255634331867,
-0.529748711727747));
#63709=CARTESIAN_POINT('Ctrl Pts',(-0.0819920957220178,-0.429442820686423,
-0.528934859067974));
#63710=CARTESIAN_POINT('Ctrl Pts',(-0.0601003545798103,-0.433622538331684,
-0.528122458082049));
#63711=CARTESIAN_POINT('Ctrl Pts',(-0.0378453166231203,-0.436132214901088,
-0.527310057096123));
#63712=CARTESIAN_POINT('Ctrl Pts',(-0.0155045831831506,-0.436924991160172,
-0.526497656110197));
#63713=CARTESIAN_POINT('Ctrl Pts',(0.00681246718488999,-0.437716927009195,
-0.525686116338208));
#63714=CARTESIAN_POINT('Ctrl Pts',(0.029214322223221,-0.436795522814159,
-0.524874576566219));
#63715=CARTESIAN_POINT('Ctrl Pts',(0.0514190471355656,-0.434165776624172,
-0.52406303679423));
#63716=CARTESIAN_POINT('Ctrl Pts',(0.0736344546586686,-0.431534765273052,
-0.523251106593467));
#63717=CARTESIAN_POINT('Ctrl Pts',(0.0956518298188783,-0.427193835658177,
-0.522439176392705));
#63718=CARTESIAN_POINT('Ctrl Pts',(0.11719430442358,-0.421199875368777,
-0.521627246191943));
#63719=CARTESIAN_POINT('Ctrl Pts',(0.138742081080045,-0.415204439840886,
-0.520815116158245));
#63720=CARTESIAN_POINT('Ctrl Pts',(0.15981404383523,-0.407555385787585,
-0.520002986124546));
#63721=CARTESIAN_POINT('Ctrl Pts',(0.180149075836899,-0.398359323318924,
-0.519190856090848));
#63722=CARTESIAN_POINT('Ctrl Pts',(0.200527815297379,-0.389143495131599,
-0.518376980491173));
#63723=CARTESIAN_POINT('Ctrl Pts',(0.220165830000383,-0.378374358729374,
-0.517563104891498));
#63724=CARTESIAN_POINT('Ctrl Pts',(0.238826165613217,-0.366204727739127,
-0.516749229291823));
#63725=CARTESIAN_POINT('Ctrl Pts',(0.247958915804214,-0.360248661242976,
-0.516350901914835));
#63726=CARTESIAN_POINT('Ctrl Pts',(0.256857931630922,-0.353957788076334,
-0.515952574537847));
#63727=CARTESIAN_POINT('Ctrl Pts',(0.265498334026349,-0.347353529749207,
-0.515554247160858));
#63728=CARTESIAN_POINT('Ctrl Pts',(0.283152162037289,-0.333859894231881,
-0.514740395828064));
#63729=CARTESIAN_POINT('Ctrl Pts',(0.299825141677166,-0.318978397252585,
-0.51392654449527));
#63730=CARTESIAN_POINT('Ctrl Pts',(0.315292491492751,-0.302877012677247,
-0.513112693162475));
#63731=CARTESIAN_POINT('Ctrl Pts',(0.330732251724026,-0.286804348633387,
-0.512300293521162));
#63732=CARTESIAN_POINT('Ctrl Pts',(0.344970120595746,-0.269516587985787,
-0.511487893879849));
#63733=CARTESIAN_POINT('Ctrl Pts',(0.357815460872545,-0.251220890772579,
-0.510675494238536));
#63734=CARTESIAN_POINT('Ctrl Pts',(0.370647183769643,-0.232944588877088,
-0.509863955824262));
#63735=CARTESIAN_POINT('Ctrl Pts',(0.382088876941243,-0.213663038361432,
-0.509052417409989));
#63736=CARTESIAN_POINT('Ctrl Pts',(0.391991011714252,-0.193615306045873,
-0.508240878995716));
#63737=CARTESIAN_POINT('Ctrl Pts',(0.401897910330637,-0.173557928915436,
-0.507428950156349));
#63738=CARTESIAN_POINT('Ctrl Pts',(0.410263437270949,-0.152734266903474,
-0.506617021316982));
#63739=CARTESIAN_POINT('Ctrl Pts',(0.416984324671081,-0.131407431215295,
-0.505805092477615));
#63740=CARTESIAN_POINT('Ctrl Pts',(0.423706866192026,-0.110075346642452,
-0.50499296380922));
#63741=CARTESIAN_POINT('Ctrl Pts',(0.428783777419164,-0.0882405335351049,
-0.504180835140825));
#63742=CARTESIAN_POINT('Ctrl Pts',(0.432162060346666,-0.0661800090429443,
-0.503368706472431));
#63743=CARTESIAN_POINT('Ctrl Pts',(0.4355476045219,-0.0440720678788024,
-0.502554832222752));
#63744=CARTESIAN_POINT('Ctrl Pts',(0.437227170701727,-0.0217381609663,-0.501740957973073));
#63745=CARTESIAN_POINT('Ctrl Pts',(0.437199666812554,0.000539758271596754,
-0.500927083723394));
#63746=CARTESIAN_POINT('Ctrl Pts',(0.437186205549979,0.0114432679023959,
-0.500528748240405));
#63747=CARTESIAN_POINT('Ctrl Pts',(0.436764624756656,0.0223333862276293,
-0.500130412757415));
#63748=CARTESIAN_POINT('Ctrl Pts',(0.435939317411843,0.0331775757778652,
-0.499732077274425));
#63749=CARTESIAN_POINT('Ctrl Pts',(0.434253107340928,0.0553336631378791,
-0.49891822615915));
#63750=CARTESIAN_POINT('Ctrl Pts',(0.430868685109664,0.0774242171171006,
-0.498104375043875));
#63751=CARTESIAN_POINT('Ctrl Pts',(0.425804304059114,0.0991692222654455,
-0.4972905239286));
#63752=CARTESIAN_POINT('Ctrl Pts',(0.42074895656677,0.120875439896079,-0.496478124515191));
#63753=CARTESIAN_POINT('Ctrl Pts',(0.414019704841125,0.142236630434071,
-0.495665725101782));
#63754=CARTESIAN_POINT('Ctrl Pts',(0.405686267894861,0.16298003571462,-0.494853325688373));
#63755=CARTESIAN_POINT('Ctrl Pts',(0.397361665348452,0.183701450604199,
-0.494041787511606));
#63756=CARTESIAN_POINT('Ctrl Pts',(0.387436493343025,0.203805709481093,
-0.49323024933484));
#63757=CARTESIAN_POINT('Ctrl Pts',(0.376029631492862,0.223037118523673,
-0.492418711158074));
#63758=CARTESIAN_POINT('Ctrl Pts',(0.364617282049137,0.242277779379574,
-0.491606782567911));
#63759=CARTESIAN_POINT('Ctrl Pts',(0.351722167742822,0.260644126579765,
-0.490794853977749));
#63760=CARTESIAN_POINT('Ctrl Pts',(0.337508546981797,0.277906136517775,
-0.489982925387587));
#63761=CARTESIAN_POINT('Ctrl Pts',(0.323291428136882,0.295172394772234,
-0.489170796975411));
#63762=CARTESIAN_POINT('Ctrl Pts',(0.30775563583115,0.311333242542577,-0.488358668563235));
#63763=CARTESIAN_POINT('Ctrl Pts',(0.291104494176897,0.326193214935585,
-0.487546540151059));
#63764=CARTESIAN_POINT('Ctrl Pts',(0.274417562854466,0.341085127089369,
-0.486732666164495));
#63765=CARTESIAN_POINT('Ctrl Pts',(0.256611061717959,0.354670141411213,
-0.485918792177932));
#63766=CARTESIAN_POINT('Ctrl Pts',(0.237920753444391,0.366793613740007,
-0.485104918191369));
#63767=CARTESIAN_POINT('Ctrl Pts',(0.228773096405688,0.37272724337087,-0.484706581256909));
#63768=CARTESIAN_POINT('Ctrl Pts',(0.219414145616143,0.378311447305482,
-0.484308244322449));
#63769=CARTESIAN_POINT('Ctrl Pts',(0.209873572367088,0.383532167649438,
-0.48390990738799));
#63770=CARTESIAN_POINT('Ctrl Pts',(0.190381206986412,0.394198632424477,
-0.483096064354828));
#63771=CARTESIAN_POINT('Ctrl Pts',(0.170017884048308,0.403405803602295,
-0.482282221321667));
#63772=CARTESIAN_POINT('Ctrl Pts',(0.149028282021272,0.411016314953297,
-0.481468378288506));
#63773=CARTESIAN_POINT('Ctrl Pts',(0.128075969059305,0.41861330585486,-0.480655981087704));
#63774=CARTESIAN_POINT('Ctrl Pts',(0.106500231687055,0.424618973788685,
-0.479843583886902));
#63775=CARTESIAN_POINT('Ctrl Pts',(0.0845677300764937,0.428943048701934,
-0.4790311866861));
#63776=CARTESIAN_POINT('Ctrl Pts',(0.0626556115000823,0.433263105023587,
-0.478219544488999));
#63777=CARTESIAN_POINT('Ctrl Pts',(0.0403880794136098,0.435904501921364,
-0.477407902291897));
#63778=CARTESIAN_POINT('Ctrl Pts',(0.0180444028609421,0.436827471120341,
-0.476596260094796));
#63779=CARTESIAN_POINT('Ctrl Pts',(0.00895914354067751,0.437202763633081,
-0.476266234737575));
#63780=CARTESIAN_POINT('Ctrl Pts',(-0.000138609858056261,0.437294532845896,
-0.475936209380354));
#63781=CARTESIAN_POINT('Ctrl Pts',(-0.00922985932074711,0.43710256198851,
-0.475606184023132));
#63782=CARTESIAN_POINT('Ctrl Pts',(-0.0092298593207472,0.43710256198851,
-0.57559571443739));
#63783=CARTESIAN_POINT('Ctrl Pts',(-0.0315292904518787,0.436631687118007,
-0.574783656190821));
#63784=CARTESIAN_POINT('Ctrl Pts',(-0.0538297205441489,0.434449229488396,
-0.573971597944252));
#63785=CARTESIAN_POINT('Ctrl Pts',(-0.0758498132990062,0.430570140421402,
-0.573159539697683));
#63786=CARTESIAN_POINT('Ctrl Pts',(-0.0987604173441071,0.42653417769141,
-0.572314641124557));
#63787=CARTESIAN_POINT('Ctrl Pts',(-0.121366684075482,0.42066129074851,
-0.57146974255143));
#63788=CARTESIAN_POINT('Ctrl Pts',(-0.1433594617347,0.41302772876786,-0.570624843978303));
#63789=CARTESIAN_POINT('Ctrl Pts',(-0.164494584018402,0.405691853853778,
-0.56981289403105));
#63790=CARTESIAN_POINT('Ctrl Pts',(-0.185062535112171,0.396730542173786,
-0.569000944083796));
#63791=CARTESIAN_POINT('Ctrl Pts',(-0.204806602463167,0.386261693140148,
-0.568188994136542));
#63792=CARTESIAN_POINT('Ctrl Pts',(-0.224560290384027,0.375787743015042,
-0.567376648555448));
#63793=CARTESIAN_POINT('Ctrl Pts',(-0.243488685069747,0.363805166334551,
-0.566564302974354));
#63794=CARTESIAN_POINT('Ctrl Pts',(-0.261361799646781,0.35047660362055,
-0.56575195739326));
#63795=CARTESIAN_POINT('Ctrl Pts',(-0.279271495348444,0.337120761172417,
-0.56493794917442));
#63796=CARTESIAN_POINT('Ctrl Pts',(-0.296121069562384,0.32241391337574,
-0.564123940955579));
#63797=CARTESIAN_POINT('Ctrl Pts',(-0.311714809764689,0.306557853224092,
-0.563309932736738));
#63798=CARTESIAN_POINT('Ctrl Pts',(-0.313561365287305,0.304680234701524,
-0.563213540764546));
#63799=CARTESIAN_POINT('Ctrl Pts',(-0.315390357015224,0.302786539933061,
-0.563117148792354));
#63800=CARTESIAN_POINT('Ctrl Pts',(-0.317201497937629,0.300877133903732,
-0.563020756820161));
#63801=CARTESIAN_POINT('Ctrl Pts',(-0.332303636588417,0.284955614910453,
-0.562216995549647));
#63802=CARTESIAN_POINT('Ctrl Pts',(-0.346252502632818,0.267842840736493,
-0.561413234279134));
#63803=CARTESIAN_POINT('Ctrl Pts',(-0.358854735651147,0.249734095991607,
-0.56060947300862));
#63804=CARTESIAN_POINT('Ctrl Pts',(-0.371487447422678,0.231581554884516,
-0.55980376782536));
#63805=CARTESIAN_POINT('Ctrl Pts',(-0.382766470990126,0.212428739913962,
-0.558998062642099));
#63806=CARTESIAN_POINT('Ctrl Pts',(-0.392536209756225,0.192507568760859,
-0.558192357458839));
#63807=CARTESIAN_POINT('Ctrl Pts',(-0.402256949762855,0.172686309457707,
-0.557390693177329));
#63808=CARTESIAN_POINT('Ctrl Pts',(-0.410483164408189,0.152105037054788,
-0.556589028895819));
#63809=CARTESIAN_POINT('Ctrl Pts',(-0.417106810099915,0.131018124579286,
-0.555787364614309));
#63810=CARTESIAN_POINT('Ctrl Pts',(-0.423780536920521,0.109771774774175,
-0.554979638980174));
#63811=CARTESIAN_POINT('Ctrl Pts',(-0.428827075457434,0.0880128079590822,
-0.554171913346038));
#63812=CARTESIAN_POINT('Ctrl Pts',(-0.432186891185448,0.0660176573914703,
-0.553364187711903));
#63813=CARTESIAN_POINT('Ctrl Pts',(-0.435546706913462,0.0440225068238584,
-0.552556462077768));
#63814=CARTESIAN_POINT('Ctrl Pts',(-0.43721973946023,0.021791931740694,
-0.551748736443633));
#63815=CARTESIAN_POINT('Ctrl Pts',(-0.437199823825906,-0.000392487702464365,
-0.550941010809498));
#63816=CARTESIAN_POINT('',(-0.43719997630689,0.00014393489640635,-0.57065898919245));
#63817=CARTESIAN_POINT('Ctrl Pts',(-0.00922985932074836,0.43710256198851,
-0.595330810493319));
#63818=CARTESIAN_POINT('Ctrl Pts',(-0.0268631581577466,0.436730217184842,
-0.59468736400291));
#63819=CARTESIAN_POINT('Ctrl Pts',(-0.0444436751027457,0.435289819211557,
-0.5940439175125));
#63820=CARTESIAN_POINT('Ctrl Pts',(-0.0618348607888011,0.432805140902034,
-0.593400471022091));
#63821=CARTESIAN_POINT('Ctrl Pts',(-0.0838331401374778,0.4296622472241,
-0.592586569319385));
#63822=CARTESIAN_POINT('Ctrl Pts',(-0.105654017097476,0.424828934836601,
-0.59177266761668));
#63823=CARTESIAN_POINT('Ctrl Pts',(-0.127019260290177,0.418341902653005,
-0.590958765913974));
#63824=CARTESIAN_POINT('Ctrl Pts',(-0.148346413599656,0.411866435528422,
-0.590146315232468));
#63825=CARTESIAN_POINT('Ctrl Pts',(-0.169218852447682,0.403743253256097,
-0.589333864550962));
#63826=CARTESIAN_POINT('Ctrl Pts',(-0.189368984193052,0.394059929231192,
-0.588521413869456));
#63827=CARTESIAN_POINT('Ctrl Pts',(-0.209497768427388,0.384386863941518,
-0.587709823916808));
#63828=CARTESIAN_POINT('Ctrl Pts',(-0.228905111152579,0.373157221535593,
-0.58689823396416));
#63829=CARTESIAN_POINT('Ctrl Pts',(-0.247343690691476,0.360506502958157,
-0.586086644011512));
#63830=CARTESIAN_POINT('Ctrl Pts',(-0.26579114352254,0.347849696410559,
-0.585274663493271));
#63831=CARTESIAN_POINT('Ctrl Pts',(-0.283268301333048,0.333770836892071,
-0.584462682975029));
#63832=CARTESIAN_POINT('Ctrl Pts',(-0.299556449929447,0.318449012097175,
-0.583650702456787));
#63833=CARTESIAN_POINT('Ctrl Pts',(-0.315848610034954,0.303123413783186,
-0.582838521960799));
#63834=CARTESIAN_POINT('Ctrl Pts',(-0.330950678613554,0.286554753730788,
-0.582026341464811));
#63835=CARTESIAN_POINT('Ctrl Pts',(-0.3446810005753,0.268958821834142,-0.581214160968823));
#63836=CARTESIAN_POINT('Ctrl Pts',(-0.358440822655247,0.251325084409538,
-0.580400235472194));
#63837=CARTESIAN_POINT('Ctrl Pts',(-0.370822612161444,0.232660262061621,
-0.579586309975564));
#63838=CARTESIAN_POINT('Ctrl Pts',(-0.381687584035801,0.21320982198978,
-0.578772384478935));
#63839=CARTESIAN_POINT('Ctrl Pts',(-0.38700079840824,0.20369812155143,-0.578374356697842));
#63840=CARTESIAN_POINT('Ctrl Pts',(-0.391951981037456,0.193998917752201,
-0.577976328916749));
#63841=CARTESIAN_POINT('Ctrl Pts',(-0.396529087440907,0.184142669724542,
-0.577578301135656));
#63842=CARTESIAN_POINT('Ctrl Pts',(-0.406675666486683,0.162293232352492,
-0.576695948839841));
#63843=CARTESIAN_POINT('Ctrl Pts',(-0.415031602930839,0.13956203722299,
-0.575813596544027));
#63844=CARTESIAN_POINT('Ctrl Pts',(-0.421462353738376,0.116246825252598,
-0.574931244248212));
#63845=CARTESIAN_POINT('Ctrl Pts',(-0.427857489738203,0.0930607376746569,
-0.574053778599118));
#63846=CARTESIAN_POINT('Ctrl Pts',(-0.432348472496993,0.0692975505394903,
-0.573176312950024));
#63847=CARTESIAN_POINT('Ctrl Pts',(-0.434849789863832,0.0452714065982187,
-0.57229884730093));
#63848=CARTESIAN_POINT('Ctrl Pts',(-0.436407991627485,0.0303042615412165,
-0.571752227931437));
#63849=CARTESIAN_POINT('Ctrl Pts',(-0.437195007874429,0.0152354700883076,
-0.571205608561943));
#63850=CARTESIAN_POINT('Ctrl Pts',(-0.437199976306891,0.000143934896406404,
-0.57065898919245));
#63851=CARTESIAN_POINT('Ctrl Pts',(-0.437199976306908,0.000143934842618929,
-0.570658989190502));
#63852=CARTESIAN_POINT('Ctrl Pts',(-0.437207536200571,-0.022819131431466,
-0.56982726089721));
#63853=CARTESIAN_POINT('Ctrl Pts',(-0.435401621291541,-0.0457679489929577,
-0.568995532603917));
#63854=CARTESIAN_POINT('Ctrl Pts',(-0.431814986033601,-0.0684080246520904,
-0.568163804310625));
#63855=CARTESIAN_POINT('Ctrl Pts',(-0.428225091115235,-0.0910686764092512,
-0.56733132011337));
#63856=CARTESIAN_POINT('Ctrl Pts',(-0.422851404212316,-0.113419377779202,
-0.566498835916116));
#63857=CARTESIAN_POINT('Ctrl Pts',(-0.415777657420984,-0.135176845611661,
-0.565666351718861));
#63858=CARTESIAN_POINT('Ctrl Pts',(-0.408683321630454,-0.156997641196864,
-0.564831444475238));
#63859=CARTESIAN_POINT('Ctrl Pts',(-0.399879295855431,-0.178221136303188,
-0.563996537231616));
#63860=CARTESIAN_POINT('Ctrl Pts',(-0.38949786065506,-0.198583122508261,
-0.563161629987993));
#63861=CARTESIAN_POINT('Ctrl Pts',(-0.383672425477592,-0.210009040835808,
-0.562693130408403));
#63862=CARTESIAN_POINT('Ctrl Pts',(-0.377351137911915,-0.221164130691169,
-0.562224630828812));
#63863=CARTESIAN_POINT('Ctrl Pts',(-0.370563342659814,-0.232005709146963,
-0.561756131249221));
#63864=CARTESIAN_POINT('Ctrl Pts',(-0.35877222017527,-0.250838684325242,
-0.560942297637313));
#63865=CARTESIAN_POINT('Ctrl Pts',(-0.345508001174671,-0.268824352225785,
-0.560128464025405));
#63866=CARTESIAN_POINT('Ctrl Pts',(-0.330916986010361,-0.285723272362996,
-0.559314630413496));
#63867=CARTESIAN_POINT('Ctrl Pts',(-0.316352005050509,-0.302592040386936,
-0.558502248894565));
#63868=CARTESIAN_POINT('Ctrl Pts',(-0.300465347420246,-0.318377337669999,
-0.557689867375634));
#63869=CARTESIAN_POINT('Ctrl Pts',(-0.283445509763087,-0.33287006923895,
-0.556877485856702));
#63870=CARTESIAN_POINT('Ctrl Pts',(-0.266443722409415,-0.347347430614106,
-0.556065965904917));
#63871=CARTESIAN_POINT('Ctrl Pts',(-0.248311664896186,-0.360534464973568,
-0.555254445953133));
#63872=CARTESIAN_POINT('Ctrl Pts',(-0.229273430822636,-0.372260035350047,
-0.554442926001348));
#63873=CARTESIAN_POINT('Ctrl Pts',(-0.210226044304049,-0.383991242679931,
-0.553631015919274));
#63874=CARTESIAN_POINT('Ctrl Pts',(-0.190272210438616,-0.394259191281616,
-0.552819105837201));
#63875=CARTESIAN_POINT('Ctrl Pts',(-0.169664271032002,-0.402936564654015,
-0.552007195755127));
#63876=CARTESIAN_POINT('Ctrl Pts',(-0.149051264462849,-0.411616071653674,
-0.551195086037357));
#63877=CARTESIAN_POINT('Ctrl Pts',(-0.127784503651842,-0.418703976275056,
-0.550382976319586));
#63878=CARTESIAN_POINT('Ctrl Pts',(-0.106134857200167,-0.424121718480792,
-0.549570866601815));
#63879=CARTESIAN_POINT('Ctrl Pts',(-0.0844386762296176,-0.429551105774012,
-0.548757011306578));
#63880=CARTESIAN_POINT('Ctrl Pts',(-0.062358672049308,-0.433303036707379,
-0.547943156011342));
#63881=CARTESIAN_POINT('Ctrl Pts',(-0.0401754613602373,-0.435350172050606,
-0.547129300716105));
#63882=CARTESIAN_POINT('Ctrl Pts',(-0.0293150275399613,-0.436352406498445,
-0.546730854264999));
#63883=CARTESIAN_POINT('Ctrl Pts',(-0.0184299106066175,-0.436946818404209,
-0.546332407813893));
#63884=CARTESIAN_POINT('Ctrl Pts',(-0.00755294417326473,-0.437134753862371,
-0.545933961362787));
#63885=CARTESIAN_POINT('Ctrl Pts',(0.0146641498154526,-0.43751862741419,
-0.545120101882027));
#63886=CARTESIAN_POINT('Ctrl Pts',(0.0369740900129726,-0.43620552516262,
-0.544306242401266));
#63887=CARTESIAN_POINT('Ctrl Pts',(0.0590963723883364,-0.433187556112291,
-0.543492382920506));
#63888=CARTESIAN_POINT('Ctrl Pts',(0.0811791982123437,-0.430174969809041,
-0.542679975011869));
#63889=CARTESIAN_POINT('Ctrl Pts',(0.103074322004255,-0.425463593101464,
-0.541867567103232));
#63890=CARTESIAN_POINT('Ctrl Pts',(0.124503674974381,-0.419097452769489,
-0.541055159194595));
#63891=CARTESIAN_POINT('Ctrl Pts',(0.145910313274123,-0.412738060414434,
-0.540243612421518));
#63892=CARTESIAN_POINT('Ctrl Pts',(0.16685147056835,-0.404727562698576,
-0.539432065648441));
#63893=CARTESIAN_POINT('Ctrl Pts',(0.187061492127124,-0.395160522020069,
-0.538620518875363));
#63894=CARTESIAN_POINT('Ctrl Pts',(0.207281237447412,-0.385588878297392,
-0.537808581638216));
#63895=CARTESIAN_POINT('Ctrl Pts',(0.226768489566447,-0.374459484778317,
-0.536996644401068));
#63896=CARTESIAN_POINT('Ctrl Pts',(0.24527892815776,-0.3619144752587,-0.53618470716392));
#63897=CARTESIAN_POINT('Ctrl Pts',(0.263793923186711,-0.349366377721841,
-0.535372570064334));
#63898=CARTESIAN_POINT('Ctrl Pts',(0.281331051587131,-0.33540239783538,
-0.534560432964749));
#63899=CARTESIAN_POINT('Ctrl Pts',(0.297676764826116,-0.320206782693086,
-0.533748295865163));
#63900=CARTESIAN_POINT('Ctrl Pts',(0.314057609401525,-0.304978508084671,
-0.532934413264402));
#63901=CARTESIAN_POINT('Ctrl Pts',(0.329241435602004,-0.288513835581878,
-0.532120530663641));
#63902=CARTESIAN_POINT('Ctrl Pts',(0.343052318357026,-0.271033110283356,
-0.53130664806288));
#63903=CARTESIAN_POINT('Ctrl Pts',(0.349810878789107,-0.262478657941508,
-0.530908362534038));
#63904=CARTESIAN_POINT('Ctrl Pts',(0.356241286735471,-0.253681362361846,
-0.530510077005196));
#63905=CARTESIAN_POINT('Ctrl Pts',(0.362326789425417,-0.244669445711289,
-0.530111791476353));
#63906=CARTESIAN_POINT('Ctrl Pts',(0.374761829137925,-0.226254608491577,
-0.52929793983247));
#63907=CARTESIAN_POINT('Ctrl Pts',(0.385824970639398,-0.206836713406551,
-0.528484088188586));
#63908=CARTESIAN_POINT('Ctrl Pts',(0.395356659951971,-0.186646595017487,
-0.527670236544703));
#63909=CARTESIAN_POINT('Ctrl Pts',(0.404871347717123,-0.166492489473992,
-0.526857836557169));
#63910=CARTESIAN_POINT('Ctrl Pts',(0.412859653188187,-0.145569510876561,
-0.526045436569635));
#63911=CARTESIAN_POINT('Ctrl Pts',(0.419206871783939,-0.124134760035713,
-0.525233036582102));
#63912=CARTESIAN_POINT('Ctrl Pts',(0.425547361943917,-0.102722731327747,
-0.524421497787712));
#63913=CARTESIAN_POINT('Ctrl Pts',(0.430249990105675,-0.0808006821067508,
-0.523609958993323));
#63914=CARTESIAN_POINT('Ctrl Pts',(0.433249183383256,-0.0586428605862762,
-0.522798420198933));
#63915=CARTESIAN_POINT('Ctrl Pts',(0.436249819722372,-0.0364743778322752,
-0.521986490932737));
#63916=CARTESIAN_POINT('Ctrl Pts',(0.437545269348742,-0.0140706027309854,
-0.521174561666541));
#63917=CARTESIAN_POINT('Ctrl Pts',(0.437121469958561,0.00828616324160506,
-0.520362632400345));
#63918=CARTESIAN_POINT('Ctrl Pts',(0.436697566250218,0.0306484323291283,
-0.519550503277869));
#63919=CARTESIAN_POINT('Ctrl Pts',(0.434553616100216,0.0529629546957005,
-0.518738374155393));
#63920=CARTESIAN_POINT('Ctrl Pts',(0.430727637927697,0.0749502630097212,
-0.517926245032917));
#63921=CARTESIAN_POINT('Ctrl Pts',(0.426893436074222,0.0969848315538128,
-0.517112370293897));
#63922=CARTESIAN_POINT('Ctrl Pts',(0.421370158290273,0.118690085595842,
-0.516298495554876));
#63923=CARTESIAN_POINT('Ctrl Pts',(0.414246596892501,0.139798415452329,
-0.515484620815855));
#63924=CARTESIAN_POINT('Ctrl Pts',(0.410760126576244,0.150129422846104,
-0.515086287740543));
#63925=CARTESIAN_POINT('Ctrl Pts',(0.406891073807587,0.160317716194181,
-0.514687954665231));
#63926=CARTESIAN_POINT('Ctrl Pts',(0.402653968465716,0.170333853589971,
-0.514289621589919));
#63927=CARTESIAN_POINT('Ctrl Pts',(0.393996981173336,0.190798195908118,
-0.513475772489442));
#63928=CARTESIAN_POINT('Ctrl Pts',(0.383751155681082,0.210659396133888,
-0.512661923388965));
#63929=CARTESIAN_POINT('Ctrl Pts',(0.372023001995696,0.22965784547041,-0.511848074288487));
#63930=CARTESIAN_POINT('Ctrl Pts',(0.360315769066053,0.248622405251188,
-0.511035676937254));
#63931=CARTESIAN_POINT('Ctrl Pts',(0.347131780986945,0.266726637689673,
-0.51022327958602));
#63932=CARTESIAN_POINT('Ctrl Pts',(0.332624019768573,0.283734209204664,
-0.509410882234786));
#63933=CARTESIAN_POINT('Ctrl Pts',(0.318131639202835,0.300723749850129,
-0.508599346160581));
#63934=CARTESIAN_POINT('Ctrl Pts',(0.302318712512743,0.316618378059953,
-0.507787810086375));
#63935=CARTESIAN_POINT('Ctrl Pts',(0.285379384357789,0.331213597220237,
-0.506976274012169));
#63936=CARTESIAN_POINT('Ctrl Pts',(0.268431907791513,0.345815837193151,
-0.506164347560631));
#63937=CARTESIAN_POINT('Ctrl Pts',(0.250357477215184,0.359116938197219,
-0.505352421109092));
#63938=CARTESIAN_POINT('Ctrl Pts',(0.23138507344878,0.370951193265506,-0.504540494657554));
#63939=CARTESIAN_POINT('Ctrl Pts',(0.212408000959996,0.382788360503076,
-0.503728368407443));
#63940=CARTESIAN_POINT('Ctrl Pts',(0.192533138946753,0.393157611381695,
-0.502916242157332));
#63941=CARTESIAN_POINT('Ctrl Pts',(0.172015488466205,0.401938442709494,
-0.502104115907221));
#63942=CARTESIAN_POINT('Ctrl Pts',(0.151453737659898,0.410738147422545,
-0.501290244085305));
#63943=CARTESIAN_POINT('Ctrl Pts',(0.130247116519065,0.417942379376124,
-0.500476372263389));
#63944=CARTESIAN_POINT('Ctrl Pts',(0.108668369482998,0.423479663589536,
-0.499662500441473));
#63945=CARTESIAN_POINT('Ctrl Pts',(0.0981066513195151,0.42618988745728,
-0.499264150862143));
#63946=CARTESIAN_POINT('Ctrl Pts',(0.087455965752906,0.428501551984591,
-0.498865801282813));
#63947=CARTESIAN_POINT('Ctrl Pts',(0.0767489199084235,0.430410784359419,
-0.498467451703484));
#63948=CARTESIAN_POINT('Ctrl Pts',(0.05487165141627,0.434311840718447,-0.497653520314069));
#63949=CARTESIAN_POINT('Ctrl Pts',(0.0326336448370843,0.436551803539617,
-0.496839588924654));
#63950=CARTESIAN_POINT('Ctrl Pts',(0.0103106826073552,0.437078402376702,
-0.496025657535238));
#63951=CARTESIAN_POINT('Ctrl Pts',(0.00380198288178817,0.437231942649321,
-0.495788339792351));
#63952=CARTESIAN_POINT('Ctrl Pts',(-0.00271386094603355,0.437240153834367,
-0.495551022049464));
#63953=CARTESIAN_POINT('Ctrl Pts',(-0.00922985932074758,0.43710256198851,
-0.495313704306577));
#63954=CARTESIAN_POINT('Origin',(0.,0.,-0.920658989190502));
#63955=CARTESIAN_POINT('',(-0.00922985932074681,0.43710256198851,-0.375613721612844));
#63956=CARTESIAN_POINT('',(-0.0092298593207473,0.43710256198851,-0.39532387974855));
#63957=CARTESIAN_POINT('',(-0.00922985932074702,0.43710256198851,-0.920658989190502));
#63958=CARTESIAN_POINT('',(-0.437199950177151,0.000208722535621865,-0.450941010807471));
#63959=CARTESIAN_POINT('Ctrl Pts',(-0.437199950177151,0.000208722535622156,
-0.450941010807471));
#63960=CARTESIAN_POINT('Ctrl Pts',(-0.437210447586036,-0.0217796393252642,
-0.450136498703844));
#63961=CARTESIAN_POINT('Ctrl Pts',(-0.435557844346497,-0.0438345863239729,
-0.449331986600217));
#63962=CARTESIAN_POINT('Ctrl Pts',(-0.432238247625148,-0.0656805701097482,
-0.44852747449659));
#63963=CARTESIAN_POINT('Ctrl Pts',(-0.428924107663845,-0.0874906434216002,
-0.447724284851645));
#63964=CARTESIAN_POINT('Ctrl Pts',(-0.423948466443405,-0.1090917095392,
-0.446921095206699));
#63965=CARTESIAN_POINT('Ctrl Pts',(-0.417359317587333,-0.130211520316123,
-0.446117905561754));
#63966=CARTESIAN_POINT('Ctrl Pts',(-0.410745398879746,-0.151410724439345,
-0.445311696575665));
#63967=CARTESIAN_POINT('Ctrl Pts',(-0.402505957615879,-0.172124316795769,
-0.444505487589576));
#63968=CARTESIAN_POINT('Ctrl Pts',(-0.39274073871354,-0.192089958495344,
-0.443699278603487));
#63969=CARTESIAN_POINT('Ctrl Pts',(-0.383014546323265,-0.211975807886681,
-0.442896291616315));
#63970=CARTESIAN_POINT('Ctrl Pts',(-0.371775107128368,-0.231119027356013,
-0.442093304629142));
#63971=CARTESIAN_POINT('Ctrl Pts',(-0.359167827505802,-0.24928359690273,
-0.44129031764197));
#63972=CARTESIAN_POINT('Ctrl Pts',(-0.346484667498001,-0.267557494914912,
-0.440482497656422));
#63973=CARTESIAN_POINT('Ctrl Pts',(-0.332417586681563,-0.28484031772645,
-0.439674677670875));
#63974=CARTESIAN_POINT('Ctrl Pts',(-0.317156271461288,-0.300924807007953,
-0.438866857685328));
#63975=CARTESIAN_POINT('Ctrl Pts',(-0.301894956241013,-0.317009296289457,
-0.438059037699781));
#63976=CARTESIAN_POINT('Ctrl Pts',(-0.285440002767781,-0.331894998055556,
-0.437251217714234));
#63977=CARTESIAN_POINT('Ctrl Pts',(-0.268014769370086,-0.34541558071329,
-0.436443397728686));
#63978=CARTESIAN_POINT('Ctrl Pts',(-0.250459433934599,-0.359037112111036,
-0.435629546315962));
#63979=CARTESIAN_POINT('Ctrl Pts',(-0.231812813534221,-0.371355830785756,
-0.434815694903237));
#63980=CARTESIAN_POINT('Ctrl Pts',(-0.212294725853223,-0.382197317330858,
-0.434001843490512));
#63981=CARTESIAN_POINT('Ctrl Pts',(-0.1928114532553,-0.393019465544209,
-0.433189443772493));
#63982=CARTESIAN_POINT('Ctrl Pts',(-0.172460390531698,-0.402369219853268,
-0.432377044054474));
#63983=CARTESIAN_POINT('Ctrl Pts',(-0.151490520190107,-0.410115181738656,
-0.431564644336455));
#63984=CARTESIAN_POINT('Ctrl Pts',(-0.13054288015175,-0.417852932076774,
-0.430753105848943));
#63985=CARTESIAN_POINT('Ctrl Pts',(-0.10897839299455,-0.423989992562469,
-0.429941567361431));
#63986=CARTESIAN_POINT('Ctrl Pts',(-0.0870663892354181,-0.428442859510468,
-0.429130028873919));
#63987=CARTESIAN_POINT('Ctrl Pts',(-0.0651438439397747,-0.432897868666,
-0.428318099967407));
#63988=CARTESIAN_POINT('Ctrl Pts',(-0.0428741455502252,-0.435666904852043,
-0.427506171060895));
#63989=CARTESIAN_POINT('Ctrl Pts',(-0.0205380549729165,-0.436717332261876,
-0.426694242154384));
#63990=CARTESIAN_POINT('Ctrl Pts',(0.00180353278951352,-0.437768018194743,
-0.425882113422236));
#63991=CARTESIAN_POINT('Ctrl Pts',(0.0242108292959832,-0.437099251179971,
-0.425069984690088));
#63992=CARTESIAN_POINT('Ctrl Pts',(0.0464024694007817,-0.434730549689701,
-0.42425785595794));
#63993=CARTESIAN_POINT('Ctrl Pts',(0.0686418078214144,-0.432356756954652,
-0.423443981650766));
#63994=CARTESIAN_POINT('Ctrl Pts',(0.0906638584377974,-0.428275858908475,
-0.422630107343592));
#63995=CARTESIAN_POINT('Ctrl Pts',(0.112195741892854,-0.422558818983952,
-0.421816233036417));
#63996=CARTESIAN_POINT('Ctrl Pts',(0.122734106495398,-0.419760724181995,
-0.421417897971696));
#63997=CARTESIAN_POINT('Ctrl Pts',(0.133155278346947,-0.416571469487715,
-0.421019562906974));
#63998=CARTESIAN_POINT('Ctrl Pts',(0.143428921514978,-0.413003613147694,
-0.420621227842253));
#63999=CARTESIAN_POINT('Ctrl Pts',(0.164419343064774,-0.405714007368978,
-0.4198073762426));
#64000=CARTESIAN_POINT('Ctrl Pts',(0.184912629682327,-0.396799260557487,
-0.418993524642946));
#64001=CARTESIAN_POINT('Ctrl Pts',(0.204642716959909,-0.386348545222143,
-0.418179673043293));
#64002=CARTESIAN_POINT('Ctrl Pts',(0.224337611028023,-0.375916471173517,
-0.417367273137665));
#64003=CARTESIAN_POINT('Ctrl Pts',(0.243271356699597,-0.363954149047342,
-0.416554873232037));
#64004=CARTESIAN_POINT('Ctrl Pts',(0.261198052034453,-0.350598656034799,
-0.415742473326409));
#64005=CARTESIAN_POINT('Ctrl Pts',(0.279105743162667,-0.337257321267503,
-0.41493093465122));
#64006=CARTESIAN_POINT('Ctrl Pts',(0.296007915887002,-0.322526150683547,
-0.41411939597603));
#64007=CARTESIAN_POINT('Ctrl Pts',(0.311687723668804,-0.306585392532259,
-0.413307857300841));
#64008=CARTESIAN_POINT('Ctrl Pts',(0.327375074729211,-0.290636965563753,
-0.412495928208727));
#64009=CARTESIAN_POINT('Ctrl Pts',(0.341838370981948,-0.273478285563776,
-0.411683999116614));
#64010=CARTESIAN_POINT('Ctrl Pts',(0.354897175683285,-0.255326917288459,
-0.4108720700245));
#64011=CARTESIAN_POINT('Ctrl Pts',(0.367959194300396,-0.237171081761341,
-0.410059941107688));
#64012=CARTESIAN_POINT('Ctrl Pts',(0.379615641078203,-0.218022670618517,
-0.409247812190875));
#64013=CARTESIAN_POINT('Ctrl Pts',(0.389729470148362,-0.198128191073044,
-0.408435683274062));
#64014=CARTESIAN_POINT('Ctrl Pts',(0.399865037643893,-0.178190950803033,
-0.407621808786534));
#64015=CARTESIAN_POINT('Ctrl Pts',(0.408451086733716,-0.157505099989189,
-0.406807934299006));
#64016=CARTESIAN_POINT('Ctrl Pts',(0.415398323941052,-0.136338081499503,
-0.405994059811478));
#64017=CARTESIAN_POINT('Ctrl Pts',(0.418798504796817,-0.125978324247186,
-0.405595725859591));
#64018=CARTESIAN_POINT('Ctrl Pts',(0.421806886383809,-0.115503537983901,
-0.405197391907705));
#64019=CARTESIAN_POINT('Ctrl Pts',(0.424417456202221,-0.104945999784821,
-0.404799057955819));
#64020=CARTESIAN_POINT('Ctrl Pts',(0.429751209670126,-0.0833754960638666,
-0.403985206863895));
#64021=CARTESIAN_POINT('Ctrl Pts',(0.433451576961043,-0.0613356638242659,
-0.403171355771971));
#64022=CARTESIAN_POINT('Ctrl Pts',(0.435448244719041,-0.0390981607125717,
-0.402357504680048));
#64023=CARTESIAN_POINT('Ctrl Pts',(0.437441350953927,-0.0169003233795044,
-0.401545105281558));
#64024=CARTESIAN_POINT('Ctrl Pts',(0.437736671263043,0.00549378516313112,
-0.400732705883068));
#64025=CARTESIAN_POINT('Ctrl Pts',(0.436315043346417,0.0278032902659854,
-0.399920306484578));
#64026=CARTESIAN_POINT('Ctrl Pts',(0.434894922503936,0.0500891449621915,
-0.399108768314342));
#64027=CARTESIAN_POINT('Ctrl Pts',(0.431761484426021,0.0722898620470738,
-0.398297230144107));
#64028=CARTESIAN_POINT('Ctrl Pts',(0.426947598401813,0.094125385624304,
-0.397485691973871));
#64029=CARTESIAN_POINT('Ctrl Pts',(0.422131396447059,0.11597141413576,-0.396673763377683));
#64030=CARTESIAN_POINT('Ctrl Pts',(0.415633267298273,0.137451195365861,
-0.395861834781494));
#64031=CARTESIAN_POINT('Ctrl Pts',(0.407537213848898,0.158294849342224,
-0.395049906185305));
#64032=CARTESIAN_POINT('Ctrl Pts',(0.399439167825586,0.179143633289868,
-0.394237777759932));
#64033=CARTESIAN_POINT('Ctrl Pts',(0.38974270292394,0.1993553229584,-0.393425649334559));
#64034=CARTESIAN_POINT('Ctrl Pts',(0.378579742042501,0.218680632235764,
-0.392613520909186));
#64035=CARTESIAN_POINT('Ctrl Pts',(0.367392787543437,0.238047479245474,
-0.391799646898648));
#64036=CARTESIAN_POINT('Ctrl Pts',(0.354733443520658,0.256523547104739,
-0.390985772888111));
#64037=CARTESIAN_POINT('Ctrl Pts',(0.340777218881838,0.273888165299561,
-0.390171898877574));
#64038=CARTESIAN_POINT('Ctrl Pts',(0.333946579630962,0.282386985409414,
-0.38977356194151));
#64039=CARTESIAN_POINT('Ctrl Pts',(0.326805888618687,0.290620077775586,
-0.389375225005447));
#64040=CARTESIAN_POINT('Ctrl Pts',(0.319378925732149,0.298564803347914,
-0.388976888069383));
#64041=CARTESIAN_POINT('Ctrl Pts',(0.304203718720093,0.314797933505676,
-0.388162982633519));
#64042=CARTESIAN_POINT('Ctrl Pts',(0.287744340900112,0.329917556773789,
-0.387349077197655));
#64043=CARTESIAN_POINT('Ctrl Pts',(0.270190222122802,0.343716574911992,
-0.386535171761791));
#64044=CARTESIAN_POINT('Ctrl Pts',(0.252668522721909,0.357490108685591,
-0.385722769466417));
#64045=CARTESIAN_POINT('Ctrl Pts',(0.234056618747682,0.369947398846978,
-0.384910367171043));
#64046=CARTESIAN_POINT('Ctrl Pts',(0.214579520855051,0.380919242398723,
-0.384097964875668));
#64047=CARTESIAN_POINT('Ctrl Pts',(0.195116095478011,0.391883383945638,
-0.383286132869724));
#64048=CARTESIAN_POINT('Ctrl Pts',(0.174789283585532,0.401363765400864,
-0.382474300863779));
#64049=CARTESIAN_POINT('Ctrl Pts',(0.153852054252127,0.409235122395916,
-0.381662468857834));
#64050=CARTESIAN_POINT('Ctrl Pts',(0.132923776607731,0.41710311400108,-0.380850983949757));
#64051=CARTESIAN_POINT('Ctrl Pts',(0.111386269345724,0.42336319726535,-0.380039499041679));
#64052=CARTESIAN_POINT('Ctrl Pts',(0.0895111269731423,0.427938778504587,
-0.379228014133602));
#64053=CARTESIAN_POINT('Ctrl Pts',(0.0676112186894509,0.432519539981572,
-0.378415610504047));
#64054=CARTESIAN_POINT('Ctrl Pts',(0.0453736167109743,0.435411863787432,
-0.377603206874493));
#64055=CARTESIAN_POINT('Ctrl Pts',(0.023079508171655,0.436590398775047,
-0.376790803244939));
#64056=CARTESIAN_POINT('Ctrl Pts',(0.0123122882369146,0.437159587060376,
-0.376398442700907));
#64057=CARTESIAN_POINT('Ctrl Pts',(0.00153195052704815,0.437329808405186,
-0.376006082156876));
#64058=CARTESIAN_POINT('Ctrl Pts',(-0.00922985932074681,0.43710256198851,
-0.375613721612844));
#64059=CARTESIAN_POINT('Ctrl Pts',(-0.00922985932074711,0.43710256198851,
-0.475606184023132));
#64060=CARTESIAN_POINT('Ctrl Pts',(-0.031596657038163,0.436630264604921,
-0.474794237278421));
#64061=CARTESIAN_POINT('Ctrl Pts',(-0.0539235984025056,0.43443692052174,
-0.47398229053371));
#64062=CARTESIAN_POINT('Ctrl Pts',(-0.0759302021839514,0.430555971270059,
-0.473170343788999));
#64063=CARTESIAN_POINT('Ctrl Pts',(-0.0988896108466164,0.426506991211468,
-0.472323242741092));
#64064=CARTESIAN_POINT('Ctrl Pts',(-0.121499442488184,0.420620914447263,
-0.471476141693185));
#64065=CARTESIAN_POINT('Ctrl Pts',(-0.143455413350369,0.412994412045096,
-0.470629040645277));
#64066=CARTESIAN_POINT('Ctrl Pts',(-0.165411384212554,0.405367909642929,
-0.46978193959737));
#64067=CARTESIAN_POINT('Ctrl Pts',(-0.186712719534122,0.39600139295843,
-0.468934838549463));
#64068=CARTESIAN_POINT('Ctrl Pts',(-0.207081768033953,0.385046726187786,
-0.468087737501556));
#64069=CARTESIAN_POINT('Ctrl Pts',(-0.226651309261429,0.374522041983556,
-0.467273886089646));
#64070=CARTESIAN_POINT('Ctrl Pts',(-0.24547239624558,0.362471566139285,
-0.466460034677735));
#64071=CARTESIAN_POINT('Ctrl Pts',(-0.263296463456217,0.349025518166579,
-0.465646183265825));
#64072=CARTESIAN_POINT('Ctrl Pts',(-0.281088737272656,0.335603454366427,
-0.464833783548326));
#64073=CARTESIAN_POINT('Ctrl Pts',(-0.297886923090229,0.320791141461004,
-0.464021383830827));
#64074=CARTESIAN_POINT('Ctrl Pts',(-0.313469956409651,0.30476290198863,
-0.463208984113328));
#64075=CARTESIAN_POINT('Ctrl Pts',(-0.329036470054283,0.28875165415698,
-0.462397445626044));
#64076=CARTESIAN_POINT('Ctrl Pts',(-0.343389872413706,0.271527529831524,
-0.461585907138759));
#64077=CARTESIAN_POINT('Ctrl Pts',(-0.356344630186733,0.253302871158383,
-0.460774368651475));
#64078=CARTESIAN_POINT('Ctrl Pts',(-0.369305620306502,0.235069444865338,
-0.459962439744753));
#64079=CARTESIAN_POINT('Ctrl Pts',(-0.380866191846791,0.215835095032773,
-0.459150510838031));
#64080=CARTESIAN_POINT('Ctrl Pts',(-0.390882676100084,0.195843237117948,
-0.458338581931309));
#64081=CARTESIAN_POINT('Ctrl Pts',(-0.400901625535766,0.175846458956176,
-0.457526453198701));
#64082=CARTESIAN_POINT('Ctrl Pts',(-0.409375438908169,0.15509245518468,
-0.456714324466092));
#64083=CARTESIAN_POINT('Ctrl Pts',(-0.416207877534535,0.133846339801273,
-0.455902195733484));
#64084=CARTESIAN_POINT('Ctrl Pts',(-0.423055001685896,0.112554558386221,
-0.455088321425474));
#64085=CARTESIAN_POINT('Ctrl Pts',(-0.428253534660455,0.090769249199721,
-0.454274447117464));
#64086=CARTESIAN_POINT('Ctrl Pts',(-0.431757704996032,0.0687686278513655,
-0.453460572809453));
#64087=CARTESIAN_POINT('Ctrl Pts',(-0.433472753503982,0.0580008485472618,
-0.453062237744676));
#64088=CARTESIAN_POINT('Ctrl Pts',(-0.434782720481834,0.0471815993014252,
-0.452663902679899));
#64089=CARTESIAN_POINT('Ctrl Pts',(-0.435686785767368,0.0363437024489768,
-0.452265567615122));
#64090=CARTESIAN_POINT('Ctrl Pts',(-0.436688861601316,0.0243308592390448,
-0.451824048679914));
#64091=CARTESIAN_POINT('Ctrl Pts',(-0.437194189162464,0.0122760091762199,
-0.451382529744706));
#64092=CARTESIAN_POINT('Ctrl Pts',(-0.437199950177124,0.00020872259101247,
-0.450941010809498));
#64093=CARTESIAN_POINT('',(-0.43719982366506,-0.000392666831192225,-0.470658989187641));
#64094=CARTESIAN_POINT('Ctrl Pts',(-0.00922985932074758,0.43710256198851,
-0.495313704306577));
#64095=CARTESIAN_POINT('Ctrl Pts',(-0.03152725504041,0.436631730097763,
-0.494501615763862));
#64096=CARTESIAN_POINT('Ctrl Pts',(-0.0538264166591165,0.434449611184395,
-0.493689527221147));
#64097=CARTESIAN_POINT('Ctrl Pts',(-0.0758460144531191,0.430570809613909,
-0.492877438678432));
#64098=CARTESIAN_POINT('Ctrl Pts',(-0.0989662333703342,0.426498131162421,
-0.492024758939984));
#64099=CARTESIAN_POINT('Ctrl Pts',(-0.121777335796485,0.420554526014737,
-0.491172079201535));
#64100=CARTESIAN_POINT('Ctrl Pts',(-0.143961542459546,0.412818258187145,
-0.490319399463087));
#64101=CARTESIAN_POINT('Ctrl Pts',(-0.165085803368755,0.405451623782063,
-0.489507460161377));
#64102=CARTESIAN_POINT('Ctrl Pts',(-0.185641063095161,0.396460216974159,
-0.488695520859668));
#64103=CARTESIAN_POINT('Ctrl Pts',(-0.205370664093565,0.385962084057189,
-0.487883581557959));
#64104=CARTESIAN_POINT('Ctrl Pts',(-0.225109510264207,0.375459031778341,
-0.487071261786381));
#64105=CARTESIAN_POINT('Ctrl Pts',(-0.244021317172783,0.363448221097851,
-0.486258942014804));
#64106=CARTESIAN_POINT('Ctrl Pts',(-0.261876166526046,0.35009243551614,
-0.485446622243226));
#64107=CARTESIAN_POINT('Ctrl Pts',(-0.27976768974906,0.336709217143978,
-0.48463263396642));
#64108=CARTESIAN_POINT('Ctrl Pts',(-0.296597391328691,0.321975988816443,
-0.483818645689614));
#64109=CARTESIAN_POINT('Ctrl Pts',(-0.3121696267946,0.306094697939903,-0.483004657412808));
#64110=CARTESIAN_POINT('Ctrl Pts',(-0.314461339323845,0.303757502784972,
-0.482884865547555));
#64111=CARTESIAN_POINT('Ctrl Pts',(-0.316725888252609,0.301395502024436,
-0.482765073682303));
#64112=CARTESIAN_POINT('Ctrl Pts',(-0.318962724860187,0.299009398096054,
-0.48264528181705));
#64113=CARTESIAN_POINT('Ctrl Pts',(-0.333977798397273,0.282992347127554,
-0.48184116243711));
#64114=CARTESIAN_POINT('Ctrl Pts',(-0.347831425387404,0.265789959998062,
-0.48103704305717));
#64115=CARTESIAN_POINT('Ctrl Pts',(-0.360331303178404,0.247598852884567,
-0.48023292367723));
#64116=CARTESIAN_POINT('Ctrl Pts',(-0.372811195416129,0.229436830802655,
-0.479430089971516));
#64117=CARTESIAN_POINT('Ctrl Pts',(-0.383941167054413,0.210289786234671,
-0.478627256265802));
#64118=CARTESIAN_POINT('Ctrl Pts',(-0.393568659859785,0.190387893460095,
-0.477824422560088));
#64119=CARTESIAN_POINT('Ctrl Pts',(-0.403186140154464,0.170506698484859,
-0.477022423794605));
#64120=CARTESIAN_POINT('Ctrl Pts',(-0.411303899013268,0.149872859957529,
-0.476220425029121));
#64121=CARTESIAN_POINT('Ctrl Pts',(-0.41781511838112,0.12874147292994,-0.475418426263638));
#64122=CARTESIAN_POINT('Ctrl Pts',(-0.424331811700911,0.107592320843235,
-0.474615753261511));
#64123=CARTESIAN_POINT('Ctrl Pts',(-0.429239034539328,0.0859454832553259,
-0.473813080259383));
#64124=CARTESIAN_POINT('Ctrl Pts',(-0.432479564362781,0.0640723529190212,
-0.473010407257255));
#64125=CARTESIAN_POINT('Ctrl Pts',(-0.435643924923276,0.0427133546250252,
-0.472226601235004));
#64126=CARTESIAN_POINT('Ctrl Pts',(-0.43721916236399,0.0211392701264403,
-0.471442795212753));
#64127=CARTESIAN_POINT('Ctrl Pts',(-0.437199823665131,-0.000392666752592153,
-0.470658989190502));
#64128=CARTESIAN_POINT('Ctrl Pts',(-0.43719982366506,-0.000392666831191846,
-0.470658989187641));
#64129=CARTESIAN_POINT('Ctrl Pts',(-0.437173552585976,-0.0296431922912459,
-0.469594210940398));
#64130=CARTESIAN_POINT('Ctrl Pts',(-0.434207981134181,-0.0587635782881525,
-0.468529432693157));
#64131=CARTESIAN_POINT('Ctrl Pts',(-0.428402952386622,-0.08726253713035,
-0.467464654445915));
#64132=CARTESIAN_POINT('Ctrl Pts',(-0.427237084359252,-0.0929861995568984,
-0.467250806940815));
#64133=CARTESIAN_POINT('Ctrl Pts',(-0.425956834269805,-0.0986848733356714,
-0.467036959435715));
#64134=CARTESIAN_POINT('Ctrl Pts',(-0.424563234051596,-0.104354685048875,
-0.466823111930615));
#64135=CARTESIAN_POINT('Ctrl Pts',(-0.419259533671851,-0.12593259680828,
-0.466009260813785));
#64136=CARTESIAN_POINT('Ctrl Pts',(-0.41229146880438,-0.147166837152214,
-0.465195409696954));
#64137=CARTESIAN_POINT('Ctrl Pts',(-0.40372305330094,-0.167784195421876,
-0.464381558580123));
#64138=CARTESIAN_POINT('Ctrl Pts',(-0.39516992165499,-0.188364777607852,
-0.463569159165125));
#64139=CARTESIAN_POINT('Ctrl Pts',(-0.385022325946846,-0.208329987179689,
-0.462756759750126));
#64140=CARTESIAN_POINT('Ctrl Pts',(-0.373393853815011,-0.227422228318109,
-0.461944360335128));
#64141=CARTESIAN_POINT('Ctrl Pts',(-0.361777709198173,-0.246494229489809,
-0.461132822156744));
#64142=CARTESIAN_POINT('Ctrl Pts',(-0.348684151388529,-0.264694477016946,
-0.46032128397836));
#64143=CARTESIAN_POINT('Ctrl Pts',(-0.334272456697672,-0.281790284951954,
-0.459509745799976));
#64144=CARTESIAN_POINT('Ctrl Pts',(-0.319853828853012,-0.298894317309442,
-0.458697817208173));
#64145=CARTESIAN_POINT('Ctrl Pts',(-0.304116244236127,-0.314892289514549,
-0.45788588861637));
#64146=CARTESIAN_POINT('Ctrl Pts',(-0.287259523413783,-0.329584293023933,
-0.457073960024566));
#64147=CARTESIAN_POINT('Ctrl Pts',(-0.270398654019511,-0.344279912351244,
-0.456261831610733));
#64148=CARTESIAN_POINT('Ctrl Pts',(-0.252418660021591,-0.35766847690647,
-0.4554497031969));
#64149=CARTESIAN_POINT('Ctrl Pts',(-0.233552218507466,-0.369590585959979,
-0.454637574783067));
#64150=CARTESIAN_POINT('Ctrl Pts',(-0.214645225799104,-0.381538320182898,
-0.453823700794849));
#64151=CARTESIAN_POINT('Ctrl Pts',(-0.194848612001848,-0.392012964846112,
-0.453009826806631));
#64152=CARTESIAN_POINT('Ctrl Pts',(-0.174420344756774,-0.400900715059138,
-0.452195952818412));
#64153=CARTESIAN_POINT('Ctrl Pts',(-0.164422073193806,-0.405250674805973,
-0.451797615893668));
#64154=CARTESIAN_POINT('Ctrl Pts',(-0.154272792737645,-0.409221240741445,
-0.451399278968925));
#64155=CARTESIAN_POINT('Ctrl Pts',(-0.144004081235465,-0.412803421240098,
-0.451000942044181));
#64156=CARTESIAN_POINT('Ctrl Pts',(-0.123023833918062,-0.420122258932769,
-0.450187090452869));
#64157=CARTESIAN_POINT('Ctrl Pts',(-0.101424225607706,-0.425858497932171,
-0.449373238861556));
#64158=CARTESIAN_POINT('Ctrl Pts',(-0.0794691881014299,-0.429916838635683,
-0.448559387270244));
#64159=CARTESIAN_POINT('Ctrl Pts',(-0.0575533124497425,-0.433967940355956,
-0.447746987370266));
#64160=CARTESIAN_POINT('Ctrl Pts',(-0.0352839517474037,-0.436346901387538,
-0.446934587470287));
#64161=CARTESIAN_POINT('Ctrl Pts',(-0.012938976963878,-0.43700849290961,
-0.446122187570308));
#64162=CARTESIAN_POINT('Ctrl Pts',(0.00938230983974245,-0.437669383076373,
-0.445310648898086));
#64163=CARTESIAN_POINT('Ctrl Pts',(0.0317783408244336,-0.436616469221204,
-0.444499110225864));
#64164=CARTESIAN_POINT('Ctrl Pts',(0.0539672160245315,-0.433856404348906,
-0.443687571553642));
#64165=CARTESIAN_POINT('Ctrl Pts',(0.0761667660106505,-0.431095011644455,
-0.442875642460473));
#64166=CARTESIAN_POINT('Ctrl Pts',(0.0981582487386274,-0.426624897012567,
-0.442063713367304));
#64167=CARTESIAN_POINT('Ctrl Pts',(0.119665135370166,-0.420504572361395,
-0.441251784274134));
#64168=CARTESIAN_POINT('Ctrl Pts',(0.141177315144382,-0.414382741413558,
-0.44043965535397));
#64169=CARTESIAN_POINT('Ctrl Pts',(0.162203982046089,-0.406610117993494,
-0.439627526433805));
#64170=CARTESIAN_POINT('Ctrl Pts',(0.182484650225093,-0.397294843198632,
-0.438815397513641));
#64171=CARTESIAN_POINT('Ctrl Pts',(0.202808909279719,-0.387959546332437,
-0.438001523019295));
#64172=CARTESIAN_POINT('Ctrl Pts',(0.222383338673432,-0.37707532065262,
-0.437187648524949));
#64173=CARTESIAN_POINT('Ctrl Pts',(0.240971885936293,-0.364796368112823,
-0.436373774030604));
#64174=CARTESIAN_POINT('Ctrl Pts',(0.250069664093788,-0.358786689968868,
-0.435975440072985));
#64175=CARTESIAN_POINT('Ctrl Pts',(0.258931738409619,-0.352443572121148,
-0.435577106115366));
#64176=CARTESIAN_POINT('Ctrl Pts',(0.267533354777696,-0.345788582925162,
-0.435178772157747));
#64177=CARTESIAN_POINT('Ctrl Pts',(0.28510764763195,-0.332191518830764,
-0.434364920745939));
#64178=CARTESIAN_POINT('Ctrl Pts',(0.301692959607839,-0.317212376336345,
-0.433551069334132));
#64179=CARTESIAN_POINT('Ctrl Pts',(0.317065499398493,-0.301020446300886,
-0.432737217922324));
#64180=CARTESIAN_POINT('Ctrl Pts',(0.332410618667629,-0.284857398361162,
-0.43192481820493));
#64181=CARTESIAN_POINT('Ctrl Pts',(0.346546732292667,-0.267486331847394,
-0.431112418487537));
#64182=CARTESIAN_POINT('Ctrl Pts',(0.3592844226865,-0.249115522629217,-0.430300018770144));
#64183=CARTESIAN_POINT('Ctrl Pts',(0.372008609772009,-0.230764188425222,
-0.429488480282968));
#64184=CARTESIAN_POINT('Ctrl Pts',(0.383336888246875,-0.211415784750808,
-0.428676941795792));
#64185=CARTESIAN_POINT('Ctrl Pts',(0.393121135724313,-0.191310252330675,
-0.427865403308615));
#64186=CARTESIAN_POINT('Ctrl Pts',(0.402910090261781,-0.17119504742952,
-0.427053474402004));
#64187=CARTESIAN_POINT('Ctrl Pts',(0.41115319997167,-0.150322621360285,
-0.426241545495393));
#64188=CARTESIAN_POINT('Ctrl Pts',(0.417748743659805,-0.128956687188586,
-0.425429616588782));
#64189=CARTESIAN_POINT('Ctrl Pts',(0.424345910593941,-0.107585494592584,
-0.424617487856286));
#64190=CARTESIAN_POINT('Ctrl Pts',(0.429294523396063,-0.0857212448492418,
-0.42380535912379));
#64191=CARTESIAN_POINT('Ctrl Pts',(0.432543211513634,-0.0636412615641114,
-0.422993230391294));
#64192=CARTESIAN_POINT('Ctrl Pts',(0.435798882305056,-0.0415138199461588,
-0.422179356083397));
#64193=CARTESIAN_POINT('Ctrl Pts',(0.437347277372875,-0.0191704335859931,
-0.4213654817755));
#64194=CARTESIAN_POINT('Ctrl Pts',(0.437188960185798,0.00310694249401093,
-0.420551607467603));
#64195=CARTESIAN_POINT('Ctrl Pts',(0.437111474895426,0.0140101740769806,
-0.420153272402173));
#64196=CARTESIAN_POINT('Ctrl Pts',(0.43662595656848,0.0248976182249839,
-0.419754937336743));
#64197=CARTESIAN_POINT('Ctrl Pts',(0.435736989139207,0.0357367639259372,
-0.419356602271314));
#64198=CARTESIAN_POINT('Ctrl Pts',(0.433920710848475,0.0578825753229286,
-0.418542750933284));
#64199=CARTESIAN_POINT('Ctrl Pts',(0.430406633419485,0.079952882377742,
-0.417728899595255));
#64200=CARTESIAN_POINT('Ctrl Pts',(0.425214654265534,0.101667781513332,
-0.416915048257226));
#64201=CARTESIAN_POINT('Ctrl Pts',(0.420031936227625,0.123343947018685,
-0.416102648614486));
#64202=CARTESIAN_POINT('Ctrl Pts',(0.413177367857804,0.14466526188217,-0.415290248971747));
#64203=CARTESIAN_POINT('Ctrl Pts',(0.404722268735889,0.165359381920938,
-0.414477849329007));
#64204=CARTESIAN_POINT('Ctrl Pts',(0.396276132926945,0.186031563970348,
-0.413666310917124));
#64205=CARTESIAN_POINT('Ctrl Pts',(0.386233078348518,0.206077201652903,
-0.412854772505241));
#64206=CARTESIAN_POINT('Ctrl Pts',(0.374713484125949,0.225241303526223,
-0.412043234093357));
#64207=CARTESIAN_POINT('Ctrl Pts',(0.363188347994157,0.244414624970205,
-0.411231305262148));
#64208=CARTESIAN_POINT('Ctrl Pts',(0.350185605792639,0.262704940483676,
-0.410419376430939));
#64209=CARTESIAN_POINT('Ctrl Pts',(0.335870863915565,0.279883194873526,
-0.40960744759973));
#64210=CARTESIAN_POINT('Ctrl Pts',(0.321552599003601,0.297065677044085,
-0.408795318942801));
#64211=CARTESIAN_POINT('Ctrl Pts',(0.305922173702576,0.313135023897119,
-0.407983190285872));
#64212=CARTESIAN_POINT('Ctrl Pts',(0.28918405650235,0.327896967757931,-0.407171061628943));
#64213=CARTESIAN_POINT('Ctrl Pts',(0.272409962661738,0.34269064070388,-0.406357187395717));
#64214=CARTESIAN_POINT('Ctrl Pts',(0.254523991886672,0.356170863517118,
-0.405543313162491));
#64215=CARTESIAN_POINT('Ctrl Pts',(0.235762810969417,0.368184379032841,
-0.404729438929265));
#64216=CARTESIAN_POINT('Ctrl Pts',(0.226580502015823,0.374064169413345,
-0.40433110341447));
#64217=CARTESIAN_POINT('Ctrl Pts',(0.217188956300894,0.379593301930375,
-0.403932767899674));
#64218=CARTESIAN_POINT('Ctrl Pts',(0.207617926817868,0.384757893309352,
-0.403534432384878));
#64219=CARTESIAN_POINT('Ctrl Pts',(0.188063231238235,0.395309737537622,
-0.402720587882132));
#64220=CARTESIAN_POINT('Ctrl Pts',(0.167646158475161,0.404397194139404,
-0.401906743379385));
#64221=CARTESIAN_POINT('Ctrl Pts',(0.14661219073182,0.411884335134048,-0.401092898876639));
#64222=CARTESIAN_POINT('Ctrl Pts',(0.125615611123411,0.419358167643997,
-0.40028050099245));
#64223=CARTESIAN_POINT('Ctrl Pts',(0.104004961028189,0.425237041178104,
-0.399468103108262));
#64224=CARTESIAN_POINT('Ctrl Pts',(0.0820474268363558,0.429432252805414,
-0.398655705224073));
#64225=CARTESIAN_POINT('Ctrl Pts',(0.0601107828488583,0.433623473145389,
-0.397844080248065));
#64226=CARTESIAN_POINT('Ctrl Pts',(0.0378286035179152,0.436134047399237,
-0.397032455272057));
#64227=CARTESIAN_POINT('Ctrl Pts',(0.0154803688227484,0.436925849751547,
-0.396220830296049));
#64228=CARTESIAN_POINT('Ctrl Pts',(0.00724780578029177,0.437217531079915,
-0.395921846780216));
#64229=CARTESIAN_POINT('Ctrl Pts',(-0.000993645708467723,0.437276477905706,
-0.395622863264383));
#64230=CARTESIAN_POINT('Ctrl Pts',(-0.0092298593207473,0.43710256198851,
-0.39532387974855));
#64231=CARTESIAN_POINT('Origin',(0.,0.,-0.920658989190502));
#64232=CARTESIAN_POINT('',(-0.00922985932074603,0.43710256198851,-0.275596058510812));
#64233=CARTESIAN_POINT('',(-0.00922985932074758,0.43710256198851,-0.295331813926952));
#64234=CARTESIAN_POINT('',(-0.00922985932074702,0.43710256198851,-0.920658989190502));
#64235=CARTESIAN_POINT('',(-0.437199947496373,0.000214264250231113,-0.350941010812191));
#64236=CARTESIAN_POINT('Ctrl Pts',(-0.437199947496409,0.000214264175926867,
-0.350941010809498));
#64237=CARTESIAN_POINT('Ctrl Pts',(-0.437211089295146,-0.022520258763288,
-0.350117162487918));
#64238=CARTESIAN_POINT('Ctrl Pts',(-0.43544457971145,-0.0452520109580569,
-0.349293314166337));
#64239=CARTESIAN_POINT('Ctrl Pts',(-0.431927926938213,-0.0676912544636132,
-0.348469465844757));
#64240=CARTESIAN_POINT('Ctrl Pts',(-0.428409577883707,-0.0901413216901649,
-0.347645220134362));
#64241=CARTESIAN_POINT('Ctrl Pts',(-0.423139546600431,-0.112297926406255,
-0.346820974423967));
#64242=CARTESIAN_POINT('Ctrl Pts',(-0.416196537937162,-0.133881596230103,
-0.345996728713572));
#64243=CARTESIAN_POINT('Ctrl Pts',(-0.409234442445989,-0.155524601107592,
-0.345170217092707));
#64244=CARTESIAN_POINT('Ctrl Pts',(-0.400590430497763,-0.176590881432304,
-0.344343705471842));
#64245=CARTESIAN_POINT('Ctrl Pts',(-0.390392136003001,-0.196819257561384,
-0.343517193850977));
#64246=CARTESIAN_POINT('Ctrl Pts',(-0.382138130313612,-0.213191125596992,
-0.342848255370678));
#64247=CARTESIAN_POINT('Ctrl Pts',(-0.372867007592829,-0.229014402602027,
-0.342179316890379));
#64248=CARTESIAN_POINT('Ctrl Pts',(-0.362667230495944,-0.244164534534403,
-0.341510378410081));
#64249=CARTESIAN_POINT('Ctrl Pts',(-0.350257857036033,-0.262596667249655,
-0.340696526563625));
#64250=CARTESIAN_POINT('Ctrl Pts',(-0.336404235292047,-0.280133047453723,
-0.33988267471717));
#64251=CARTESIAN_POINT('Ctrl Pts',(-0.321260540146733,-0.296539213839636,
-0.339068822870715));
#64252=CARTESIAN_POINT('Ctrl Pts',(-0.306143857926695,-0.312916115337265,
-0.338256422751787));
#64253=CARTESIAN_POINT('Ctrl Pts',(-0.289742109223225,-0.328166247186758,
-0.33744402263286));
#64254=CARTESIAN_POINT('Ctrl Pts',(-0.27225063444735,-0.342086877917022,
-0.336631622513932));
#64255=CARTESIAN_POINT('Ctrl Pts',(-0.254777703215119,-0.355992750725109,
-0.335820083658978));
#64256=CARTESIAN_POINT('Ctrl Pts',(-0.236217879135763,-0.368571455511955,
-0.335008544804023));
#64257=CARTESIAN_POINT('Ctrl Pts',(-0.21680082004648,-0.379659379480046,
-0.334197005949068));
#64258=CARTESIAN_POINT('Ctrl Pts',(-0.197374420979929,-0.390752636951906,
-0.333385076728383));
#64259=CARTESIAN_POINT('Ctrl Pts',(-0.177090575262683,-0.400353310004381,
-0.332573147507699));
#64260=CARTESIAN_POINT('Ctrl Pts',(-0.156205719281849,-0.408342519539222,
-0.331761218287014));
#64261=CARTESIAN_POINT('Ctrl Pts',(-0.135315724054299,-0.416333695021011,
-0.330949089270621));
#64262=CARTESIAN_POINT('Ctrl Pts',(-0.113825103464974,-0.422712391422751,
-0.330136960254228));
#64263=CARTESIAN_POINT('Ctrl Pts',(-0.0920071930443114,-0.427409073871984,
-0.329324831237835));
#64264=CARTESIAN_POINT('Ctrl Pts',(-0.0701423889445194,-0.43211585099644,
-0.328510956696011));
#64265=CARTESIAN_POINT('Ctrl Pts',(-0.0479495998776903,-0.435133293229205,
-0.327697082154186));
#64266=CARTESIAN_POINT('Ctrl Pts',(-0.0257102052507155,-0.436443381604036,
-0.326883207612362));
#64267=CARTESIAN_POINT('Ctrl Pts',(-0.0148256217155885,-0.437084575602048,
-0.32648487458279));
#64268=CARTESIAN_POINT('Ctrl Pts',(-0.00392990203914814,-0.437317587185639,
-0.326086541553219));
#64269=CARTESIAN_POINT('Ctrl Pts',(0.00694421185564129,-0.437144847758388,
-0.325688208523647));
#64270=CARTESIAN_POINT('Ctrl Pts',(0.0291618100177887,-0.436791912777334,
-0.324874348813205));
#64271=CARTESIAN_POINT('Ctrl Pts',(0.0514159432842557,-0.434739857967319,
-0.324060489102762));
#64272=CARTESIAN_POINT('Ctrl Pts',(0.0734260003306082,-0.430990095565373,
-0.32324662939232));
#64273=CARTESIAN_POINT('Ctrl Pts',(0.0953967989195519,-0.427247021464472,
-0.322434221330853));
#64274=CARTESIAN_POINT('Ctrl Pts',(0.117123678599569,-0.421812314603624,
-0.321621813269387));
#64275=CARTESIAN_POINT('Ctrl Pts',(0.138330183008807,-0.414739195722746,
-0.32080940520792));
#64276=CARTESIAN_POINT('Ctrl Pts',(0.159514206969538,-0.407673574866139,
-0.319997858358526));
#64277=CARTESIAN_POINT('Ctrl Pts',(0.180178266695892,-0.398973188936921,
-0.319186311509131));
#64278=CARTESIAN_POINT('Ctrl Pts',(0.200059988304416,-0.388741354990226,
-0.318374764659736));
#64279=CARTESIAN_POINT('Ctrl Pts',(0.219951272906357,-0.37850459959042,
-0.317562827460988));
#64280=CARTESIAN_POINT('Ctrl Pts',(0.239058822880429,-0.366735235436711,
-0.316750890262239));
#64281=CARTESIAN_POINT('Ctrl Pts',(0.257143164034255,-0.3535834175841,-0.315938953063491));
#64282=CARTESIAN_POINT('Ctrl Pts',(0.275231955281206,-0.340428363406001,
-0.315126816067796));
#64283=CARTESIAN_POINT('Ctrl Pts',(0.292296476518162,-0.325890624459326,
-0.314314679072101));
#64284=CARTESIAN_POINT('Ctrl Pts',(0.308129404466762,-0.310161425878458,
-0.313502542076406));
#64285=CARTESIAN_POINT('Ctrl Pts',(0.323996359718719,-0.294398422923984,
-0.312688659678217));
#64286=CARTESIAN_POINT('Ctrl Pts',(0.338625963946799,-0.277439386363242,
-0.311874777280029));
#64287=CARTESIAN_POINT('Ctrl Pts',(0.351849693310249,-0.25951037227341,
-0.31106089488184));
#64288=CARTESIAN_POINT('Ctrl Pts',(0.358320921275683,-0.250736543485635,
-0.310662609466964));
#64289=CARTESIAN_POINT('Ctrl Pts',(0.364456125959481,-0.241730884102552,
-0.310264324052088));
#64290=CARTESIAN_POINT('Ctrl Pts',(0.37023949937262,-0.232522156157885,
-0.309866038637212));
#64291=CARTESIAN_POINT('Ctrl Pts',(0.382056895684477,-0.213705597053647,
-0.309052206249676));
#64292=CARTESIAN_POINT('Ctrl Pts',(0.392469966357593,-0.193932044311778,
-0.308238373862141));
#64293=CARTESIAN_POINT('Ctrl Pts',(0.401326898651035,-0.173437482739868,
-0.307424541474605));
#64294=CARTESIAN_POINT('Ctrl Pts',(0.410168032450458,-0.152979478205733,
-0.306612160755173));
#64295=CARTESIAN_POINT('Ctrl Pts',(0.417458205930442,-0.131803645208973,
-0.305799780035741));
#64296=CARTESIAN_POINT('Ctrl Pts',(0.423091301325727,-0.110170734510135,
-0.304987399316309));
#64297=CARTESIAN_POINT('Ctrl Pts',(0.428718425496042,-0.0885607552490719,
-0.304175879741186));
#64298=CARTESIAN_POINT('Ctrl Pts',(0.432691752470204,-0.0664953421261078,
-0.303364360166062));
#64299=CARTESIAN_POINT('Ctrl Pts',(0.434954837451626,-0.0442507556707181,
-0.302552840590939));
#64300=CARTESIAN_POINT('Ctrl Pts',(0.437219012156079,-0.0219954579789519,
-0.301740930252066));
#64301=CARTESIAN_POINT('Ctrl Pts',(0.437771208707934,0.00043847537874489,
-0.300929019913194));
#64302=CARTESIAN_POINT('Ctrl Pts',(0.436606731545274,0.0227684424006747,
-0.300117109574321));
#64303=CARTESIAN_POINT('Ctrl Pts',(0.435441967537652,0.0451039099500344,
-0.29930499923806));
#64304=CARTESIAN_POINT('Ctrl Pts',(0.432559756713184,0.0673346474730818,
-0.2984928889018));
#64305=CARTESIAN_POINT('Ctrl Pts',(0.428007361644517,0.0891826125323723,
-0.297680778565539));
#64306=CARTESIAN_POINT('Ctrl Pts',(0.423445178452432,0.111077552991472,
-0.296866922107494));
#64307=CARTESIAN_POINT('Ctrl Pts',(0.417205834699874,0.132587387596294,
-0.296053065649448));
#64308=CARTESIAN_POINT('Ctrl Pts',(0.409386945720571,0.153447608888449,
-0.295239209191403));
#64309=CARTESIAN_POINT('Ctrl Pts',(0.405558983960924,0.163660329597941,
-0.294840762377861));
#64310=CARTESIAN_POINT('Ctrl Pts',(0.401353165163034,0.173717644055453,
-0.294442315564319));
#64311=CARTESIAN_POINT('Ctrl Pts',(0.396785001936018,0.183590583197054,
-0.294043868750778));
#64312=CARTESIAN_POINT('Ctrl Pts',(0.387454150385809,0.203756878689673,
-0.293230008150127));
#64313=CARTESIAN_POINT('Ctrl Pts',(0.376555297387723,0.223267664750025,
-0.292416147549476));
#64314=CARTESIAN_POINT('Ctrl Pts',(0.364203505370233,0.241867002040449,
-0.291602286948825));
#64315=CARTESIAN_POINT('Ctrl Pts',(0.351873748820917,0.260433158307072,
-0.290789878267));
#64316=CARTESIAN_POINT('Ctrl Pts',(0.338096543508109,0.278090473234571,
-0.289977469585175));
#64317=CARTESIAN_POINT('Ctrl Pts',(0.323032626525938,0.294607810826111,
-0.28916506090335));
#64318=CARTESIAN_POINT('Ctrl Pts',(0.307984683331389,0.311107633421845,
-0.288353513700233));
#64319=CARTESIAN_POINT('Ctrl Pts',(0.291653196375196,0.326469333806669,
-0.287541966497116));
#64320=CARTESIAN_POINT('Ctrl Pts',(0.274238987269211,0.340494960111831,
-0.286730419294));
#64321=CARTESIAN_POINT('Ctrl Pts',(0.256816410500093,0.354527325839693,
-0.28591848213613));
#64322=CARTESIAN_POINT('Ctrl Pts',(0.238310617794821,0.367221871584436,
-0.28510654497826));
#64323=CARTESIAN_POINT('Ctrl Pts',(0.218955961826285,0.378420568654409,
-0.28429460782039));
#64324=CARTESIAN_POINT('Ctrl Pts',(0.199596548531911,0.389622018336003,
-0.283482471090406));
#64325=CARTESIAN_POINT('Ctrl Pts',(0.17938849147353,0.399326556419703,-0.282670334360422));
#64326=CARTESIAN_POINT('Ctrl Pts',(0.158590651123122,0.407422195488101,
-0.281858197630437));
#64327=CARTESIAN_POINT('Ctrl Pts',(0.137748121701303,0.415535229948826,
-0.281044315832902));
#64328=CARTESIAN_POINT('Ctrl Pts',(0.1163139628022,0.42203224894274,-0.280230434035367));
#64329=CARTESIAN_POINT('Ctrl Pts',(0.0945631436825621,0.426850854347126,
-0.279416552237832));
#64330=CARTESIAN_POINT('Ctrl Pts',(0.0839190756782834,0.429208906396934,
-0.279018267780003));
#64331=CARTESIAN_POINT('Ctrl Pts',(0.0731993284726913,0.431165798971983,
-0.278619983322173));
#64332=CARTESIAN_POINT('Ctrl Pts',(0.0624366031354644,0.432718743052464,
-0.278221698864344));
#64333=CARTESIAN_POINT('Ctrl Pts',(0.0404381850287124,0.435892875264188,
-0.277407627357897));
#64334=CARTESIAN_POINT('Ctrl Pts',(0.0181342531020704,0.437394274199899,
-0.27659355585145));
#64335=CARTESIAN_POINT('Ctrl Pts',(-0.00419770291906552,0.437179847763141,
-0.275779484345003));
#64336=CARTESIAN_POINT('Ctrl Pts',(-0.00587497476798022,0.437163742974752,
-0.275718342400273));
#64337=CARTESIAN_POINT('Ctrl Pts',(-0.00755240007482553,0.437137983224171,
-0.275657200455542));
#64338=CARTESIAN_POINT('Ctrl Pts',(-0.00922985932074603,0.43710256198851,
-0.275596058510812));
#64339=CARTESIAN_POINT('Ctrl Pts',(-0.00922985932074681,0.43710256198851,
-0.375613721612844));
#64340=CARTESIAN_POINT('Ctrl Pts',(-0.0317120106057848,0.436627828798559,
-0.374794053802879));
#64341=CARTESIAN_POINT('Ctrl Pts',(-0.0541124227825446,0.43441512874084,
-0.373974385992914));
#64342=CARTESIAN_POINT('Ctrl Pts',(-0.0761493254630166,0.430517270538044,
-0.373154718182949));
#64343=CARTESIAN_POINT('Ctrl Pts',(-0.0980298880315945,0.426647065567484,
-0.372340865480442));
#64344=CARTESIAN_POINT('Ctrl Pts',(-0.11967720422635,0.42109345977911,-0.371527012777935));
#64345=CARTESIAN_POINT('Ctrl Pts',(-0.140814437977076,0.413902324295479,
-0.370713160075428));
#64346=CARTESIAN_POINT('Ctrl Pts',(-0.16191396871899,0.406724015818812,
-0.369900759062199));
#64347=CARTESIAN_POINT('Ctrl Pts',(-0.182504535270659,0.397914150857145,
-0.369088358048971));
#64348=CARTESIAN_POINT('Ctrl Pts',(-0.202321615710707,0.387569095538085,
-0.368275957035743));
#64349=CARTESIAN_POINT('Ctrl Pts',(-0.22211768799125,0.377235007050031,
-0.367464417251802));
#64350=CARTESIAN_POINT('Ctrl Pts',(-0.241141258078628,0.365369263937545,
-0.366652877467861));
#64351=CARTESIAN_POINT('Ctrl Pts',(-0.259149649006979,0.352115463192913,
-0.36584133768392));
#64352=CARTESIAN_POINT('Ctrl Pts',(-0.277166703195314,0.338855286469323,
-0.365029407494186));
#64353=CARTESIAN_POINT('Ctrl Pts',(-0.294167015236909,0.324206127234508,
-0.364217477304452));
#64354=CARTESIAN_POINT('Ctrl Pts',(-0.309937942529275,0.308354198578064,
-0.363405547114719));
#64355=CARTESIAN_POINT('Ctrl Pts',(-0.325712751120537,0.292498368687908,
-0.362593417105172));
#64356=CARTESIAN_POINT('Ctrl Pts',(-0.340257090489989,0.275439709384688,
-0.361781287095625));
#64357=CARTESIAN_POINT('Ctrl Pts',(-0.353396572576067,0.25739988828958,
-0.360969157086077));
#64358=CARTESIAN_POINT('Ctrl Pts',(-0.366564295920897,0.239321293424545,
-0.360155281530276));
#64359=CARTESIAN_POINT('Ctrl Pts',(-0.37832075156722,0.220257932975055,
-0.359341405974474));
#64360=CARTESIAN_POINT('Ctrl Pts',(-0.388535381537813,0.200459714888717,
-0.358527530418673));
#64361=CARTESIAN_POINT('Ctrl Pts',(-0.393534630752391,0.190770061273941,
-0.35812920304462));
#64362=CARTESIAN_POINT('Ctrl Pts',(-0.398165279852222,0.180904733858332,
-0.357730875670568));
#64363=CARTESIAN_POINT('Ctrl Pts',(-0.402416276549772,0.170894646984093,
-0.357332548296515));
#64364=CARTESIAN_POINT('Ctrl Pts',(-0.412033637771879,0.148248047096182,
-0.356431381225949));
#64365=CARTESIAN_POINT('Ctrl Pts',(-0.419751737952197,0.124749261219136,
-0.355530214155383));
#64366=CARTESIAN_POINT('Ctrl Pts',(-0.425441532179863,0.1007141633359,-0.354629047084817));
#64367=CARTESIAN_POINT('Ctrl Pts',(-0.43109173274687,0.0768463188666618,
-0.353734150979732));
#64368=CARTESIAN_POINT('Ctrl Pts',(-0.434741554040949,0.0524500065223676,
-0.352839254874646));
#64369=CARTESIAN_POINT('Ctrl Pts',(-0.436311747948595,0.0278549565076211,
-0.35194435876956));
#64370=CARTESIAN_POINT('Ctrl Pts',(-0.436898576162864,0.0186630540236529,
-0.351609909450437));
#64371=CARTESIAN_POINT('Ctrl Pts',(-0.437195424372157,0.00944356716727992,
-0.351275460131314));
#64372=CARTESIAN_POINT('Ctrl Pts',(-0.437199947496373,0.000214264250231167,
-0.350941010812191));
#64373=CARTESIAN_POINT('',(-0.437199956252192,0.000195583950560346,-0.37065898918853));
#64374=CARTESIAN_POINT('Ctrl Pts',(-0.0092298593207473,0.43710256198851,
-0.39532387974855));
#64375=CARTESIAN_POINT('Ctrl Pts',(-0.0315967145607968,0.436630263390273,
-0.394511938566279));
#64376=CARTESIAN_POINT('Ctrl Pts',(-0.0539244619775135,0.434436892463301,
-0.393699997384007));
#64377=CARTESIAN_POINT('Ctrl Pts',(-0.0759325594972625,0.430555555542133,
-0.392888056201736));
#64378=CARTESIAN_POINT('Ctrl Pts',(-0.0979513364331321,0.426672335204552,
-0.392075721025493));
#64379=CARTESIAN_POINT('Ctrl Pts',(-0.119649459095544,0.421099685297624,
-0.391263385849249));
#64380=CARTESIAN_POINT('Ctrl Pts',(-0.140758031335858,0.413921510209911,
-0.390451050673006));
#64381=CARTESIAN_POINT('Ctrl Pts',(-0.16190982507083,0.406728637232986,
-0.389637052175337));
#64382=CARTESIAN_POINT('Ctrl Pts',(-0.182469006676033,0.39792396999991,
-0.388823053677668));
#64383=CARTESIAN_POINT('Ctrl Pts',(-0.202187227238474,0.387639220334601,
-0.388009055179999));
#64384=CARTESIAN_POINT('Ctrl Pts',(-0.204583719604231,0.386389243239631,
-0.387910124286147));
#64385=CARTESIAN_POINT('Ctrl Pts',(-0.206967823593862,0.385117457043982,
-0.387811193392296));
#64386=CARTESIAN_POINT('Ctrl Pts',(-0.209339122541238,0.383824141728558,
-0.387712262498445));
#64387=CARTESIAN_POINT('Ctrl Pts',(-0.228846531848669,0.37318472772745,
-0.386898410899664));
#64388=CARTESIAN_POINT('Ctrl Pts',(-0.247596540127881,0.361023942572635,
-0.386084559300883));
#64389=CARTESIAN_POINT('Ctrl Pts',(-0.265341350695688,0.34747346317523,
-0.385270707702102));
#64390=CARTESIAN_POINT('Ctrl Pts',(-0.28305450925764,0.333947154216364,
-0.384458307797352));
#64391=CARTESIAN_POINT('Ctrl Pts',(-0.299765433088831,0.319036456730761,
-0.383645907892601));
#64392=CARTESIAN_POINT('Ctrl Pts',(-0.315254085039217,0.302916988407858,
-0.382833507987851));
#64393=CARTESIAN_POINT('Ctrl Pts',(-0.330726317368614,0.286814608438495,
-0.38202196931354));
#64394=CARTESIAN_POINT('Ctrl Pts',(-0.344978336906196,0.269506495667498,
-0.381210430639228));
#64395=CARTESIAN_POINT('Ctrl Pts',(-0.357825860337883,0.25120607809815,
-0.380398891964917));
#64396=CARTESIAN_POINT('Ctrl Pts',(-0.370679564486306,0.232896856520951,
-0.379586962873676));
#64397=CARTESIAN_POINT('Ctrl Pts',(-0.382126996289671,0.213594951382642,
-0.378775033782434));
#64398=CARTESIAN_POINT('Ctrl Pts',(-0.392025918765554,0.193544617636407,
-0.377963104691192));
#64399=CARTESIAN_POINT('Ctrl Pts',(-0.401927277475406,0.17348934928196,
-0.377150975775248));
#64400=CARTESIAN_POINT('Ctrl Pts',(-0.410279079762644,0.152685940947287,
-0.376338846859304));
#64401=CARTESIAN_POINT('Ctrl Pts',(-0.41698664526085,0.131400067253036,
-0.375526717943361));
#64402=CARTESIAN_POINT('Ctrl Pts',(-0.423708627842109,0.110068442203989,
-0.374712843456683));
#64403=CARTESIAN_POINT('Ctrl Pts',(-0.428779149029836,0.088252978039073,
-0.373898968970005));
#64404=CARTESIAN_POINT('Ctrl Pts',(-0.432154071737152,0.0662321544342359,
-0.373085094483327));
#64405=CARTESIAN_POINT('Ctrl Pts',(-0.433805857533288,0.0554545198617944,
-0.372686760526221));
#64406=CARTESIAN_POINT('Ctrl Pts',(-0.435052268808273,0.0446277950996431,
-0.372288426569115));
#64407=CARTESIAN_POINT('Ctrl Pts',(-0.435892678136593,0.033784806450657,
-0.371890092612009));
#64408=CARTESIAN_POINT('Ctrl Pts',(-0.43675847661306,0.0226142461816568,
-0.37147972480484));
#64409=CARTESIAN_POINT('Ctrl Pts',(-0.437194939423667,0.0114099837046195,
-0.371069356997671));
#64410=CARTESIAN_POINT('Ctrl Pts',(-0.437199956252168,0.000195584004442945,
-0.370658989190502));
#64411=CARTESIAN_POINT('Ctrl Pts',(-0.437199956252192,0.00019558395055889,
-0.37065898918853));
#64412=CARTESIAN_POINT('Ctrl Pts',(-0.437209797318043,-0.0218027116530455,
-0.36985400697195));
#64413=CARTESIAN_POINT('Ctrl Pts',(-0.43555503723887,-0.0438677724418389,
-0.369049024755369));
#64414=CARTESIAN_POINT('Ctrl Pts',(-0.432231672166008,-0.0657238280730574,
-0.368244042538789));
#64415=CARTESIAN_POINT('Ctrl Pts',(-0.428913828524319,-0.0875435721031573,
-0.367440397717833));
#64416=CARTESIAN_POINT('Ctrl Pts',(-0.423932935122254,-0.109154275283681,
-0.366636752896876));
#64417=CARTESIAN_POINT('Ctrl Pts',(-0.41733687497774,-0.130283432499356,
-0.36583310807592));
#64418=CARTESIAN_POINT('Ctrl Pts',(-0.410657747974787,-0.151678677754392,
-0.365019342630058));
#64419=CARTESIAN_POINT('Ctrl Pts',(-0.402322582880881,-0.172579399162873,
-0.364205577184196));
#64420=CARTESIAN_POINT('Ctrl Pts',(-0.392433908419011,-0.192716028194281,
-0.363391811738334));
#64421=CARTESIAN_POINT('Ctrl Pts',(-0.382671012325383,-0.212596530648642,
-0.362588396930498));
#64422=CARTESIAN_POINT('Ctrl Pts',(-0.371394308094424,-0.231731635324634,
-0.361784982122661));
#64423=CARTESIAN_POINT('Ctrl Pts',(-0.358749524065807,-0.249885211612367,
-0.360981567314825));
#64424=CARTESIAN_POINT('Ctrl Pts',(-0.345860380122883,-0.268389604990845,
-0.36016262654995));
#64425=CARTESIAN_POINT('Ctrl Pts',(-0.331550130208112,-0.28587345548614,
-0.359343685785075));
#64426=CARTESIAN_POINT('Ctrl Pts',(-0.316016681609745,-0.30212132818516,
-0.3585247450202));
#64427=CARTESIAN_POINT('Ctrl Pts',(-0.300483233011378,-0.31836920088418,
-0.357705804255325));
#64428=CARTESIAN_POINT('Ctrl Pts',(-0.283727222915686,-0.333380613157547,
-0.35688686349045));
#64429=CARTESIAN_POINT('Ctrl Pts',(-0.265981928594421,-0.346983362225327,
-0.356067922725575));
#64430=CARTESIAN_POINT('Ctrl Pts',(-0.248346914651699,-0.360501575286587,
-0.355254071371781));
#64431=CARTESIAN_POINT('Ctrl Pts',(-0.22962828453433,-0.372710590695404,
-0.354440220017987));
#64432=CARTESIAN_POINT('Ctrl Pts',(-0.210046876199587,-0.383437282744904,
-0.353626368664193));
#64433=CARTESIAN_POINT('Ctrl Pts',(-0.190500396005526,-0.394144841165067,
-0.352813969009587));
#64434=CARTESIAN_POINT('Ctrl Pts',(-0.170094786286069,-0.403374935974287,
-0.352001569354981));
#64435=CARTESIAN_POINT('Ctrl Pts',(-0.149079796723947,-0.410997632850539,
-0.351189169700375));
#64436=CARTESIAN_POINT('Ctrl Pts',(-0.128087085406607,-0.418612248813575,
-0.350377631280475));
#64437=CARTESIAN_POINT('Ctrl Pts',(-0.106486936500757,-0.424622580888818,
-0.349566092860576));
#64438=CARTESIAN_POINT('Ctrl Pts',(-0.0845491661335071,-0.428946708235567,
-0.348754554440676));
#64439=CARTESIAN_POINT('Ctrl Pts',(-0.0626008419783057,-0.433272915826677,
-0.347942625607154));
#64440=CARTESIAN_POINT('Ctrl Pts',(-0.0403152703163706,-0.43591114144486,
-0.347130696773632));
#64441=CARTESIAN_POINT('Ctrl Pts',(-0.01797339879321,-0.43683039836511,
-0.34631876794011));
#64442=CARTESIAN_POINT('Ctrl Pts',(0.00437397125136595,-0.437749881522174,
-0.345506639284112));
#64443=CARTESIAN_POINT('Ctrl Pts',(0.0267769527679093,-0.436949555850671,
-0.344694510628114));
#64444=CARTESIAN_POINT('Ctrl Pts',(0.0489543001086752,-0.434450591553136,
-0.343882381972117));
#64445=CARTESIAN_POINT('Ctrl Pts',(0.071179314951276,-0.431946256036789,
-0.343068507744676));
#64446=CARTESIAN_POINT('Ctrl Pts',(0.093177022140436,-0.427736120776913,
-0.342254633517235));
#64447=CARTESIAN_POINT('Ctrl Pts',(0.114674963735666,-0.421892750224774,
-0.341440759289794));
#64448=CARTESIAN_POINT('Ctrl Pts',(0.125196728244188,-0.419032822049172,
-0.341042423806243));
#64449=CARTESIAN_POINT('Ctrl Pts',(0.135599004985787,-0.415782428010782,
-0.340644088322692));
#64450=CARTESIAN_POINT('Ctrl Pts',(0.145851532189345,-0.41215430430607,
-0.340245752839141));
#64451=CARTESIAN_POINT('Ctrl Pts',(0.166798817261596,-0.404741562061054,
-0.339431900140907));
#64452=CARTESIAN_POINT('Ctrl Pts',(0.187239430905852,-0.395706621866752,
-0.338618047442673));
#64453=CARTESIAN_POINT('Ctrl Pts',(0.206907836438915,-0.385140217609337,
-0.337804194744438));
#64454=CARTESIAN_POINT('Ctrl Pts',(0.226541158947589,-0.374592660910136,
-0.336991793735514));
#64455=CARTESIAN_POINT('Ctrl Pts',(0.245404357843054,-0.362519348440181,
-0.33617939272659));
#64456=CARTESIAN_POINT('Ctrl Pts',(0.263252339930174,-0.349058799518488,
-0.335366991717666));
#64457=CARTESIAN_POINT('Ctrl Pts',(0.281081401305644,-0.335612520174361,
-0.334555451938048));
#64458=CARTESIAN_POINT('Ctrl Pts',(0.297896797365796,-0.320782330393067,
-0.33374391215843));
#64459=CARTESIAN_POINT('Ctrl Pts',(0.313482743356919,-0.304749749167116,
-0.332932372378813));
#64460=CARTESIAN_POINT('Ctrl Pts',(0.329076187247889,-0.288709455179399,
-0.332120442193377));
#64461=CARTESIAN_POINT('Ctrl Pts',(0.343438487359899,-0.271466114248043,
-0.331308512007942));
#64462=CARTESIAN_POINT('Ctrl Pts',(0.356390487247955,-0.25323834741043,
-0.330496581822506));
#64463=CARTESIAN_POINT('Ctrl Pts',(0.369345674683841,-0.235006094634032,
-0.32968445181725));
#64464=CARTESIAN_POINT('Ctrl Pts',(0.380889482304987,-0.215789534962041,
-0.328872321811993));
#64465=CARTESIAN_POINT('Ctrl Pts',(0.390886313736336,-0.195835976607004,
-0.328060191806737));
#64466=CARTESIAN_POINT('Ctrl Pts',(0.400904631792151,-0.175839531201396,
-0.327246316255148));
#64467=CARTESIAN_POINT('Ctrl Pts',(0.409369058235974,-0.155103585576575,
-0.326432440703559));
#64468=CARTESIAN_POINT('Ctrl Pts',(0.41619187118334,-0.133896102859307,
-0.32561856515197));
#64469=CARTESIAN_POINT('Ctrl Pts',(0.419531095878111,-0.1235167255336,-0.325220237752215));
#64470=CARTESIAN_POINT('Ctrl Pts',(0.422477865488116,-0.113024625635012,
-0.32482191035246));
#64471=CARTESIAN_POINT('Ctrl Pts',(0.425026357386873,-0.102452113333234,
-0.324423582952706));
#64472=CARTESIAN_POINT('Ctrl Pts',(0.430233348946519,-0.080850717485575,
-0.323609734021301));
#64473=CARTESIAN_POINT('Ctrl Pts',(0.43380423538123,-0.0587895925647821,
-0.322795885089896));
#64474=CARTESIAN_POINT('Ctrl Pts',(0.435670299321658,-0.0365408030696792,
-0.321982036158491));
#64475=CARTESIAN_POINT('Ctrl Pts',(0.437533034704557,-0.0143316994471554,
-0.321169638915277));
#64476=CARTESIAN_POINT('Ctrl Pts',(0.437696869278996,0.00806370382861299,
-0.320357241672064));
#64477=CARTESIAN_POINT('Ctrl Pts',(0.436144289949209,0.0303644256441752,
-0.319544844428851));
#64478=CARTESIAN_POINT('Ctrl Pts',(0.43459335649725,0.0526415066299919,
-0.318733308401928));
#64479=CARTESIAN_POINT('Ctrl Pts',(0.431329643147004,0.0748233933029086,
-0.317921772375005));
#64480=CARTESIAN_POINT('Ctrl Pts',(0.426387662689023,0.0966302287412781,
-0.317110236348082));
#64481=CARTESIAN_POINT('Ctrl Pts',(0.421443304411229,0.118447556476376,
-0.316298309852912));
#64482=CARTESIAN_POINT('Ctrl Pts',(0.41481920581988,0.139888770494463,-0.315486383357742));
#64483=CARTESIAN_POINT('Ctrl Pts',(0.406600952687178,0.160684489836074,
-0.314674456862573));
#64484=CARTESIAN_POINT('Ctrl Pts',(0.398380676684247,0.181485327910446,
-0.31386233051691));
#64485=CARTESIAN_POINT('Ctrl Pts',(0.388565757169535,0.201639701359637,
-0.313050204171248));
#64486=CARTESIAN_POINT('Ctrl Pts',(0.377289578154882,0.220899104153257,
-0.312238077825586));
#64487=CARTESIAN_POINT('Ctrl Pts',(0.365989161212073,0.240199904659756,
-0.31142420583009));
#64488=CARTESIAN_POINT('Ctrl Pts',(0.353221616938479,0.258601301089725,
-0.310610333834595));
#64489=CARTESIAN_POINT('Ctrl Pts',(0.339163746543061,0.275883658506397,
-0.309796461839099));
#64490=CARTESIAN_POINT('Ctrl Pts',(0.332283122866943,0.284342507128237,
-0.309398112248157));
#64491=CARTESIAN_POINT('Ctrl Pts',(0.325093993353602,0.292533795250246,
-0.308999762657214));
#64492=CARTESIAN_POINT('Ctrl Pts',(0.317620272842288,0.300435021726147,
-0.308601413066272));
#64493=CARTESIAN_POINT('Ctrl Pts',(0.302349949891085,0.316578825848198,
-0.307787504265165));
#64494=CARTESIAN_POINT('Ctrl Pts',(0.285802006571729,0.331601593610649,
-0.306973595464059));
#64495=CARTESIAN_POINT('Ctrl Pts',(0.268167087518553,0.345297340232758,
-0.306159686662952));
#64496=CARTESIAN_POINT('Ctrl Pts',(0.250564779980651,0.358967759885753,
-0.305347282989213));
#64497=CARTESIAN_POINT('Ctrl Pts',(0.231880012732739,0.371315552973588,
-0.304534879315474));
#64498=CARTESIAN_POINT('Ctrl Pts',(0.212338786939443,0.382172839905043,
-0.303722475641736));
#64499=CARTESIAN_POINT('Ctrl Pts',(0.192811611077644,0.393022320563789,
-0.302910656077514));
#64500=CARTESIAN_POINT('Ctrl Pts',(0.172429803304405,0.402383042990127,
-0.302098836513293));
#64501=CARTESIAN_POINT('Ctrl Pts',(0.151447051746655,0.410131235724915,
-0.301287016949071));
#64502=CARTESIAN_POINT('Ctrl Pts',(0.130473291938885,0.417876108122441,
-0.300475545274331));
#64503=CARTESIAN_POINT('Ctrl Pts',(0.108899770708046,0.42400957704949,-0.29966407359959));
#64504=CARTESIAN_POINT('Ctrl Pts',(0.0869985137521189,0.42845664728759,
-0.29885260192485));
#64505=CARTESIAN_POINT('Ctrl Pts',(0.0650733633028138,0.432908569121355,
-0.298040244963337));
#64506=CARTESIAN_POINT('Ctrl Pts',(0.0428204685794942,0.435670295902952,
-0.297227888001824));
#64507=CARTESIAN_POINT('Ctrl Pts',(0.0205211119096451,0.43671812873522,
-0.296415531040311));
#64508=CARTESIAN_POINT('Ctrl Pts',(0.010605030029012,0.437184079224994,
-0.296054292002525));
#64509=CARTESIAN_POINT('Ctrl Pts',(0.000679806771193227,0.437311814534476,
-0.295693052964738));
#64510=CARTESIAN_POINT('Ctrl Pts',(-0.00922985932074758,0.43710256198851,
-0.295331813926952));
#64511=CARTESIAN_POINT('Origin',(0.,0.,-0.920658989190502));
#64512=CARTESIAN_POINT('',(-0.00922985932074711,0.43710256198851,-0.175603427251549));
#64513=CARTESIAN_POINT('',(-0.00922985932074797,0.43710256198851,-0.195314102181071));
#64514=CARTESIAN_POINT('',(-0.00922985932074702,0.43710256198851,-0.920658989190502));
#64515=CARTESIAN_POINT('',(-0.437199828329094,-0.000387439040882649,-0.250941010806415));
#64516=CARTESIAN_POINT('Ctrl Pts',(-0.437199828329094,-0.00038743904088227,
-0.250941010806416));
#64517=CARTESIAN_POINT('Ctrl Pts',(-0.43717515196089,-0.028233120049581,
-0.249928536965401));
#64518=CARTESIAN_POINT('Ctrl Pts',(-0.434486254312535,-0.0559608307135708,
-0.248916063124386));
#64519=CARTESIAN_POINT('Ctrl Pts',(-0.429223229213364,-0.0831339852506318,
-0.247903589283372));
#64520=CARTESIAN_POINT('Ctrl Pts',(-0.426925233122178,-0.0949986071619341,
-0.247461512552739));
#64521=CARTESIAN_POINT('Ctrl Pts',(-0.42413710727963,-0.106757801910374,
-0.247019435822107));
#64522=CARTESIAN_POINT('Ctrl Pts',(-0.420869149183294,-0.118376514840278,
-0.246577359091474));
#64523=CARTESIAN_POINT('Ctrl Pts',(-0.414852133348964,-0.139769071786505,
-0.245763400463551));
#64524=CARTESIAN_POINT('Ctrl Pts',(-0.407182709648748,-0.160762817480468,
-0.244949441835628));
#64525=CARTESIAN_POINT('Ctrl Pts',(-0.397933943629819,-0.181086765135445,
-0.244135483207705));
#64526=CARTESIAN_POINT('Ctrl Pts',(-0.388701689625341,-0.201374428023709,
-0.243322977757059));
#64527=CARTESIAN_POINT('Ctrl Pts',(-0.377895932657817,-0.220993999659641,
-0.242510472306414));
#64528=CARTESIAN_POINT('Ctrl Pts',(-0.365638766296714,-0.239691744916292,
-0.241697966855769));
#64529=CARTESIAN_POINT('Ctrl Pts',(-0.353394619145413,-0.258369629965361,
-0.240886324425059));
#64530=CARTESIAN_POINT('Ctrl Pts',(-0.339702490091048,-0.276127022019479,
-0.24007468199435));
#64531=CARTESIAN_POINT('Ctrl Pts',(-0.324729310597089,-0.292736596344118,
-0.23926303956364));
#64532=CARTESIAN_POINT('Ctrl Pts',(-0.309748999178721,-0.309354082029776,
-0.238451010536853));
#64533=CARTESIAN_POINT('Ctrl Pts',(-0.29348688338928,-0.324822113908098,
-0.237638981510066));
#64534=CARTESIAN_POINT('Ctrl Pts',(-0.276149330728357,-0.338947469585304,
-0.236826952483278));
#64535=CARTESIAN_POINT('Ctrl Pts',(-0.258807555287566,-0.353076265671243,
-0.236014725676568));
#64536=CARTESIAN_POINT('Ctrl Pts',(-0.240390395703553,-0.365861307147297,
-0.235202498869858));
#64537=CARTESIAN_POINT('Ctrl Pts',(-0.221135719732469,-0.37715094253946,
-0.234390272063148));
#64538=CARTESIAN_POINT('Ctrl Pts',(-0.201839772608195,-0.388464776535246,
-0.233576304300786));
#64539=CARTESIAN_POINT('Ctrl Pts',(-0.181703366188955,-0.3982764850038,
-0.232762336538424));
#64540=CARTESIAN_POINT('Ctrl Pts',(-0.16098813901441,-0.406480822544775,
-0.231948368776062));
#64541=CARTESIAN_POINT('Ctrl Pts',(-0.15086612230538,-0.410489682354834,
-0.231550642252388));
#64542=CARTESIAN_POINT('Ctrl Pts',(-0.140606183717589,-0.414115518715765,
-0.231152915728714));
#64543=CARTESIAN_POINT('Ctrl Pts',(-0.130240030003468,-0.417350421809653,
-0.23075518920504));
#64544=CARTESIAN_POINT('Ctrl Pts',(-0.109020412341652,-0.423972299964116,
-0.229941039135587));
#64545=CARTESIAN_POINT('Ctrl Pts',(-0.0872341704118623,-0.428990553146929,
-0.229126889066133));
#64546=CARTESIAN_POINT('Ctrl Pts',(-0.0651484699482539,-0.432318767651141,
-0.228312738996679));
#64547=CARTESIAN_POINT('Ctrl Pts',(-0.0431020702402091,-0.435641059710425,
-0.227500037679685));
#64548=CARTESIAN_POINT('Ctrl Pts',(-0.0207579606770463,-0.437279122771291,
-0.226687336362691));
#64549=CARTESIAN_POINT('Ctrl Pts',(0.00160444992955381,-0.43719705596038,
-0.225874635045697));
#64550=CARTESIAN_POINT('Ctrl Pts',(0.0239432157696132,-0.43711507592234,
-0.225062793033778));
#64551=CARTESIAN_POINT('Ctrl Pts',(0.0462995328254728,-0.435316551808519,
-0.224250951021858));
#64552=CARTESIAN_POINT('Ctrl Pts',(0.0683917067825807,-0.43181757079045,
-0.223439109009938));
#64553=CARTESIAN_POINT('Ctrl Pts',(0.0904944859685637,-0.428316910105428,
-0.222626877277642));
#64554=CARTESIAN_POINT('Ctrl Pts',(0.112332159703595,-0.423114255294599,
-0.221814645545347));
#64555=CARTESIAN_POINT('Ctrl Pts',(0.133630135588047,-0.416277343681734,
-0.221002413813051));
#64556=CARTESIAN_POINT('Ctrl Pts',(0.154933351152798,-0.409438750067195,
-0.220189982257324));
#64557=CARTESIAN_POINT('Ctrl Pts',(0.175695933661859,-0.400965347569769,
-0.219377550701598));
#64558=CARTESIAN_POINT('Ctrl Pts',(0.195660974687255,-0.390973941566996,
-0.218565119145871));
#64559=CARTESIAN_POINT('Ctrl Pts',(0.215668795638291,-0.380961126562095,
-0.217750946759184));
#64560=CARTESIAN_POINT('Ctrl Pts',(0.234875045798112,-0.369424176900229,
-0.216936774372497));
#64561=CARTESIAN_POINT('Ctrl Pts',(0.253048763665302,-0.356525122827918,
-0.216122601985811));
#64562=CARTESIAN_POINT('Ctrl Pts',(0.261899935778643,-0.350242877855939,
-0.215726074430076));
#64563=CARTESIAN_POINT('Ctrl Pts',(0.270506665361262,-0.343638176717351,
-0.21532954687434));
#64564=CARTESIAN_POINT('Ctrl Pts',(0.278845254818156,-0.336733075098657,
-0.214933019318605));
#64565=CARTESIAN_POINT('Ctrl Pts',(0.295938302881246,-0.322578494823539,
-0.214120188251246));
#64566=CARTESIAN_POINT('Ctrl Pts',(0.312000410918705,-0.307078035278154,
-0.213307357183887));
#64567=CARTESIAN_POINT('Ctrl Pts',(0.326813749353737,-0.290407667311579,
-0.212494526116528));
#64568=CARTESIAN_POINT('Ctrl Pts',(0.341600620471756,-0.273767084657452,
-0.211683147352283));
#64569=CARTESIAN_POINT('Ctrl Pts',(0.355142637308786,-0.255961235444033,
-0.210871768588038));
#64570=CARTESIAN_POINT('Ctrl Pts',(0.367257567579701,-0.237203960876377,
-0.210060389823792));
#64571=CARTESIAN_POINT('Ctrl Pts',(0.379359676986439,-0.218466536564906,
-0.209249869717145));
#64572=CARTESIAN_POINT('Ctrl Pts',(0.390037287005823,-0.198780270088444,
-0.208439349610498));
#64573=CARTESIAN_POINT('Ctrl Pts',(0.39915046323598,-0.178389314978512,
-0.207628829503852));
#64574=CARTESIAN_POINT('Ctrl Pts',(0.408268202657258,-0.157988149616636,
-0.206817903549884));
#64575=CARTESIAN_POINT('Ctrl Pts',(0.415819633610496,-0.136882238240811,
-0.206006977595917));
#64576=CARTESIAN_POINT('Ctrl Pts',(0.421711976104694,-0.115337978176637,
-0.20519605164195));
#64577=CARTESIAN_POINT('Ctrl Pts',(0.427605824304418,-0.0937882127788037,
-0.204384918467223));
#64578=CARTESIAN_POINT('Ctrl Pts',(0.431839582023699,-0.0718005760780592,
-0.203573785292495));
#64579=CARTESIAN_POINT('Ctrl Pts',(0.434371248107624,-0.0496533867669199,
-0.202762652117767));
#64580=CARTESIAN_POINT('Ctrl Pts',(0.436908445724973,-0.0274578072203115,
-0.201949746667345));
#64581=CARTESIAN_POINT('Ctrl Pts',(0.43773609446431,-0.00510269711023237,
-0.201136841216923));
#64582=CARTESIAN_POINT('Ctrl Pts',(0.436864255439904,0.0171307419260887,
-0.200323935766501));
#64583=CARTESIAN_POINT('Ctrl Pts',(0.436430578105641,0.0281902819361774,
-0.199919573655058));
#64584=CARTESIAN_POINT('Ctrl Pts',(0.435577202005302,0.0392197681305007,
-0.199515211543615));
#64585=CARTESIAN_POINT('Ctrl Pts',(0.434310110882799,0.0501853323688408,
-0.199110849432172));
#64586=CARTESIAN_POINT('Ctrl Pts',(0.431756587431705,0.0722838420496241,
-0.198295952921602));
#64587=CARTESIAN_POINT('Ctrl Pts',(0.427504918281149,0.0942495724137049,
-0.197481056411031));
#64588=CARTESIAN_POINT('Ctrl Pts',(0.421584542938335,0.115802906507027,
-0.19666615990046));
#64589=CARTESIAN_POINT('Ctrl Pts',(0.41567478439003,0.137317589787553,-0.195852724714264));
#64590=CARTESIAN_POINT('Ctrl Pts',(0.408102393480184,0.158420649713672,
-0.195039289528069));
#64591=CARTESIAN_POINT('Ctrl Pts',(0.398947945800709,0.178841763974174,
-0.194225854341873));
#64592=CARTESIAN_POINT('Ctrl Pts',(0.389803334365754,0.199240936214769,
-0.193413293173169));
#64593=CARTESIAN_POINT('Ctrl Pts',(0.379080305967078,0.218958958286204,
-0.192600732004464));
#64594=CARTESIAN_POINT('Ctrl Pts',(0.366907889356692,0.237744486219592,
-0.19178817083576));
#64595=CARTESIAN_POINT('Ctrl Pts',(0.354730083304338,0.256538331606766,
-0.190975249898621));
#64596=CARTESIAN_POINT('Ctrl Pts',(0.341101978880221,0.274398248767588,
-0.190162328961482));
#64597=CARTESIAN_POINT('Ctrl Pts',(0.32619694664029,0.291100312611567,-0.189349408024344));
#64598=CARTESIAN_POINT('Ctrl Pts',(0.311288547867978,0.307806148875347,
-0.188536303476421));
#64599=CARTESIAN_POINT('Ctrl Pts',(0.295103144584151,0.3233530990482,-0.187723198928498));
#64600=CARTESIAN_POINT('Ctrl Pts',(0.277851824848643,0.337553260135758,
-0.186910094380575));
#64601=CARTESIAN_POINT('Ctrl Pts',(0.260564312822474,0.351783212356134,
-0.186095283985413));
#64602=CARTESIAN_POINT('Ctrl Pts',(0.242207000193842,0.364660317308267,
-0.185280473590252));
#64603=CARTESIAN_POINT('Ctrl Pts',(0.223021837114547,0.376038695043546,
-0.18446566319509));
#64604=CARTESIAN_POINT('Ctrl Pts',(0.213784259313793,0.381517337531054,
-0.184073335311972));
#64605=CARTESIAN_POINT('Ctrl Pts',(0.204355136177859,0.386649196640079,
-0.183681007428854));
#64606=CARTESIAN_POINT('Ctrl Pts',(0.19476325782855,0.391421912263493,-0.183288679545737));
#64607=CARTESIAN_POINT('Ctrl Pts',(0.17482500171414,0.401342766448193,-0.182473163175578));
#64608=CARTESIAN_POINT('Ctrl Pts',(0.15407180251471,0.409763693222663,-0.18165764680542));
#64609=CARTESIAN_POINT('Ctrl Pts',(0.132754872050416,0.416557299716231,
-0.180842130435262));
#64610=CARTESIAN_POINT('Ctrl Pts',(0.111475306657736,0.423338998135435,
-0.180028043531116));
#64611=CARTESIAN_POINT('Ctrl Pts',(0.0896346266806214,0.428498773999735,
-0.179213956626969));
#64612=CARTESIAN_POINT('Ctrl Pts',(0.0675039988359496,0.43195723184264,
-0.178399869722823));
#64613=CARTESIAN_POINT('Ctrl Pts',(0.0453962963714171,0.435412107028003,
-0.177586626140966));
#64614=CARTESIAN_POINT('Ctrl Pts',(0.0229999384184317,0.43716902774766,
-0.176773382559109));
#64615=CARTESIAN_POINT('Ctrl Pts',(0.000596477640129765,0.437199593108714,
-0.175960138977252));
#64616=CARTESIAN_POINT('Ctrl Pts',(-0.0026791203620098,0.437204062053784,
-0.175841235068684));
#64617=CARTESIAN_POINT('Ctrl Pts',(-0.00595486139123389,0.437171716856941,
-0.175722331160117));
#64618=CARTESIAN_POINT('Ctrl Pts',(-0.00922985932074711,0.43710256198851,
-0.175603427251549));
#64619=CARTESIAN_POINT('Ctrl Pts',(-0.00922985932074603,0.43710256198851,
-0.275596058510812));
#64620=CARTESIAN_POINT('Ctrl Pts',(-0.0315175128047482,0.436631935814847,
-0.274783692737513));
#64621=CARTESIAN_POINT('Ctrl Pts',(-0.053811199458999,0.434451425783461,
-0.273971326964214));
#64622=CARTESIAN_POINT('Ctrl Pts',(-0.0758295964441591,0.430573701360308,
-0.273158961190914));
#64623=CARTESIAN_POINT('Ctrl Pts',(-0.0978258595168454,0.42669987500535,
-0.272347412045317));
#64624=CARTESIAN_POINT('Ctrl Pts',(-0.119546676627676,0.421132319555819,
-0.271535862899719));
#64625=CARTESIAN_POINT('Ctrl Pts',(-0.14071744677465,0.413935309164637,
-0.270724313754122));
#64626=CARTESIAN_POINT('Ctrl Pts',(-0.161899378925678,0.406734504246444,
-0.269912336730143));
#64627=CARTESIAN_POINT('Ctrl Pts',(-0.182530002334501,0.39790274367376,
-0.269100359706165));
#64628=CARTESIAN_POINT('Ctrl Pts',(-0.202350636352501,0.387553944590605,
-0.268288382682186));
#64629=CARTESIAN_POINT('Ctrl Pts',(-0.222177114956752,0.377202093917437,
-0.267476166227433));
#64630=CARTESIAN_POINT('Ctrl Pts',(-0.241192510643821,0.365332675222146,
-0.26666394977268));
#64631=CARTESIAN_POINT('Ctrl Pts',(-0.259164041999417,0.352104869796662,
-0.265851733317928));
#64632=CARTESIAN_POINT('Ctrl Pts',(-0.277173773677142,0.338848947322146,
-0.265037790414293));
#64633=CARTESIAN_POINT('Ctrl Pts',(-0.29413466693318,0.324229339238528,
-0.264223847510659));
#64634=CARTESIAN_POINT('Ctrl Pts',(-0.309847353017181,0.308445226625809,
-0.263409904607024));
#64635=CARTESIAN_POINT('Ctrl Pts',(-0.31634892088569,0.301914104012707,
-0.263073112730652));
#64636=CARTESIAN_POINT('Ctrl Pts',(-0.322637237278018,0.295184021827159,
-0.262736320854281));
#64637=CARTESIAN_POINT('Ctrl Pts',(-0.328700221991952,0.288270713154218,
-0.262399528977909));
#64638=CARTESIAN_POINT('Ctrl Pts',(-0.343220359896925,0.2717141490118,-0.261592951900623));
#64639=CARTESIAN_POINT('Ctrl Pts',(-0.356531992844097,0.254005601113313,
-0.260786374823338));
#64640=CARTESIAN_POINT('Ctrl Pts',(-0.368448821091825,0.235349328097712,
-0.259979797746052));
#64641=CARTESIAN_POINT('Ctrl Pts',(-0.380344742409986,0.216725785719645,
-0.25917463573071));
#64642=CARTESIAN_POINT('Ctrl Pts',(-0.390850274299905,0.197158392385561,
-0.258369473715368));
#64643=CARTESIAN_POINT('Ctrl Pts',(-0.399820049116241,0.17688348799333,
-0.257564311700026));
#64644=CARTESIAN_POINT('Ctrl Pts',(-0.40878017178987,0.156630400901375,
-0.256760016098707));
#64645=CARTESIAN_POINT('Ctrl Pts',(-0.416207497594123,0.135671966911522,
-0.255955720497387));
#64646=CARTESIAN_POINT('Ctrl Pts',(-0.42200318132526,0.114267908668004,
-0.255151424896067));
#64647=CARTESIAN_POINT('Ctrl Pts',(-0.427801701475788,0.0928533752349068,
-0.254346735670846));
#64648=CARTESIAN_POINT('Ctrl Pts',(-0.43196677910013,0.0709934828957616,
-0.253542046445625));
#64649=CARTESIAN_POINT('Ctrl Pts',(-0.434449677398004,0.0489624122033488,
-0.252737357220404));
#64650=CARTESIAN_POINT('Ctrl Pts',(-0.436297241776996,0.0325687397451478,
-0.252138575083435));
#64651=CARTESIAN_POINT('Ctrl Pts',(-0.437214422054611,0.0160806372592578,
-0.251539792946467));
#64652=CARTESIAN_POINT('Ctrl Pts',(-0.437199828329169,-0.000387438956102599,
-0.250941010809498));
#64653=CARTESIAN_POINT('',(-0.437199941752427,0.000225680469443025,-0.270658989193252));
#64654=CARTESIAN_POINT('Ctrl Pts',(-0.00922985932074758,0.43710256198851,
-0.295331813926952));
#64655=CARTESIAN_POINT('Ctrl Pts',(-0.0325709355740933,0.436609691735741,
-0.294480957011248));
#64656=CARTESIAN_POINT('Ctrl Pts',(-0.0558246518002711,0.434243140628511,
-0.293630100095543));
#64657=CARTESIAN_POINT('Ctrl Pts',(-0.0786759310588921,0.430062713882541,
-0.292779243179838));
#64658=CARTESIAN_POINT('Ctrl Pts',(-0.100533583978425,0.426064061735552,
-0.291965383485719));
#64659=CARTESIAN_POINT('Ctrl Pts',(-0.122148097674547,0.420383379243374,
-0.2911515237916));
#64660=CARTESIAN_POINT('Ctrl Pts',(-0.143242906605044,0.413068165933104,
-0.29033766409748));
#64661=CARTESIAN_POINT('Ctrl Pts',(-0.164300089563836,0.405766000477875,
-0.289525256052529));
#64662=CARTESIAN_POINT('Ctrl Pts',(-0.184838721069643,0.39683527062798,
-0.288712848007577));
#64663=CARTESIAN_POINT('Ctrl Pts',(-0.204594846587949,0.386373897603932,
-0.287900439962625));
#64664=CARTESIAN_POINT('Ctrl Pts',(-0.224330029161878,0.375923614403804,
-0.287088893129882));
#64665=CARTESIAN_POINT('Ctrl Pts',(-0.243283710418694,0.363946217876189,
-0.286277346297139));
#64666=CARTESIAN_POINT('Ctrl Pts',(-0.261214058100043,0.350586730854017,
-0.285465799464396));
#64667=CARTESIAN_POINT('Ctrl Pts',(-0.279153030175122,0.337220817995707,
-0.284653862282312));
#64668=CARTESIAN_POINT('Ctrl Pts',(-0.296067100426924,0.322471899138628,
-0.283841925100227));
#64669=CARTESIAN_POINT('Ctrl Pts',(-0.311744720888325,0.306527435963341,
-0.283029987918142));
#64670=CARTESIAN_POINT('Ctrl Pts',(-0.32742619921006,0.290579049264572,
-0.28221785093914));
#64671=CARTESIAN_POINT('Ctrl Pts',(-0.341870143007703,0.273435064679692,
-0.281405713960137));
#64672=CARTESIAN_POINT('Ctrl Pts',(-0.354903466385701,0.255318173163239,
-0.280593576981134));
#64673=CARTESIAN_POINT('Ctrl Pts',(-0.367964800306894,0.237162345762387,
-0.279779694599423));
#64674=CARTESIAN_POINT('Ctrl Pts',(-0.379609082787468,0.21803004565943,
-0.278965812217711));
#64675=CARTESIAN_POINT('Ctrl Pts',(-0.389707223032687,0.198171946339918,
-0.278151929836));
#64676=CARTESIAN_POINT('Ctrl Pts',(-0.394648898968172,0.188454088482066,
-0.277753644321801));
#64677=CARTESIAN_POINT('Ctrl Pts',(-0.399221026801609,0.178562761786,-0.277355358807602));
#64678=CARTESIAN_POINT('Ctrl Pts',(-0.403412739191937,0.168528934778744,
-0.276957073293403));
#64679=CARTESIAN_POINT('Ctrl Pts',(-0.412935550646297,0.145733896890115,
-0.276052240732498));
#64680=CARTESIAN_POINT('Ctrl Pts',(-0.42053826809405,0.122091879741921,
-0.275147408171593));
#64681=CARTESIAN_POINT('Ctrl Pts',(-0.426092790488426,0.0979222849702084,
-0.274242575610688));
#64682=CARTESIAN_POINT('Ctrl Pts',(-0.431607015213754,0.0739280389075253,
-0.27334430754633));
#64683=CARTESIAN_POINT('Ctrl Pts',(-0.43510245696255,0.0494142356025085,
-0.272446039481973));
#64684=CARTESIAN_POINT('Ctrl Pts',(-0.436500945633631,0.024713649284278,
-0.271547771417616));
#64685=CARTESIAN_POINT('Ctrl Pts',(-0.436962185776802,0.0165670677599341,
-0.271251510676161));
#64686=CARTESIAN_POINT('Ctrl Pts',(-0.437195722049905,0.00840030763711254,
-0.270955249934706));
#64687=CARTESIAN_POINT('Ctrl Pts',(-0.437199941752427,0.000225680469444049,
-0.270658989193251));
#64688=CARTESIAN_POINT('Ctrl Pts',(-0.437199941752466,0.000225680393569806,
-0.270658989190502));
#64689=CARTESIAN_POINT('Ctrl Pts',(-0.437211658071991,-0.0224717907196608,
-0.269836398816264));
#64690=CARTESIAN_POINT('Ctrl Pts',(-0.435451497671837,-0.0451684701615349,
-0.269013808442026));
#64691=CARTESIAN_POINT('Ctrl Pts',(-0.431946071086998,-0.0675753777089434,
-0.268191218067787));
#64692=CARTESIAN_POINT('Ctrl Pts',(-0.428439190565981,-0.0899915789079819,
-0.267368286509994));
#64693=CARTESIAN_POINT('Ctrl Pts',(-0.42318574251998,-0.112117092405877,
-0.266545354952201));
#64694=CARTESIAN_POINT('Ctrl Pts',(-0.416263570354819,-0.133673033912822,
-0.265722423394408));
#64695=CARTESIAN_POINT('Ctrl Pts',(-0.40932251389466,-0.155287781925684,
-0.264897246806886));
#64696=CARTESIAN_POINT('Ctrl Pts',(-0.400703886039429,-0.176329206487253,
-0.264072070219364));
#64697=CARTESIAN_POINT('Ctrl Pts',(-0.390534527426051,-0.196536568831632,
-0.263246893631841));
#64698=CARTESIAN_POINT('Ctrl Pts',(-0.381858571956055,-0.213776414777793,
-0.262542896890217));
#64699=CARTESIAN_POINT('Ctrl Pts',(-0.372054857008198,-0.230409337630752,
-0.261838900148593));
#64700=CARTESIAN_POINT('Ctrl Pts',(-0.361227100237478,-0.246290117654004,
-0.261134903406969));
#64701=CARTESIAN_POINT('Ctrl Pts',(-0.348709593271618,-0.264649208901961,
-0.260321042853594));
#64702=CARTESIAN_POINT('Ctrl Pts',(-0.334753100380863,-0.2821040656358,
-0.25950718230022));
#64703=CARTESIAN_POINT('Ctrl Pts',(-0.319513172884127,-0.298421132551832,
-0.258693321746845));
#64704=CARTESIAN_POINT('Ctrl Pts',(-0.304300433255758,-0.314709089994243,
-0.257880913112031));
#64705=CARTESIAN_POINT('Ctrl Pts',(-0.287809246239468,-0.329862731700687,
-0.257068504477217));
#64706=CARTESIAN_POINT('Ctrl Pts',(-0.270236141695493,-0.343680473291011,
-0.256256095842403));
#64707=CARTESIAN_POINT('Ctrl Pts',(-0.25268167167555,-0.357483562545028,
-0.255444548685889));
#64708=CARTESIAN_POINT('Ctrl Pts',(-0.234048104169553,-0.369953102104183,
-0.254633001529375));
#64709=CARTESIAN_POINT('Ctrl Pts',(-0.214566056380477,-0.380926826896361,
-0.253821454372862));
#64710=CARTESIAN_POINT('Ctrl Pts',(-0.195074647287965,-0.391905824664393,
-0.253009517260463));
#64711=CARTESIAN_POINT('Ctrl Pts',(-0.174734557699403,-0.401387204353369,
-0.252197580148064));
#64712=CARTESIAN_POINT('Ctrl Pts',(-0.153802920495106,-0.40925359087878,
-0.251385643035665));
#64713=CARTESIAN_POINT('Ctrl Pts',(-0.132866138331588,-0.417121910948018,
-0.250573506350567));
#64714=CARTESIAN_POINT('Ctrl Pts',(-0.111338199713712,-0.4233742254396,
-0.249761369665469));
#64715=CARTESIAN_POINT('Ctrl Pts',(-0.0894928473206696,-0.427942601616665,
-0.248949232980371));
#64716=CARTESIAN_POINT('Ctrl Pts',(-0.0676005549841006,-0.432520794038206,
-0.248135351226142));
#64717=CARTESIAN_POINT('Ctrl Pts',(-0.0453901970621191,-0.435407725064112,
-0.247321469471912));
#64718=CARTESIAN_POINT('Ctrl Pts',(-0.0231432582016464,-0.436587024085476,
-0.246507587717683));
#64719=CARTESIAN_POINT('Ctrl Pts',(-0.012256398968934,-0.437164131008787,
-0.2461093029853));
#64720=CARTESIAN_POINT('Ctrl Pts',(-0.00136080249563929,-0.437333095328693,
-0.245711018252918));
#64721=CARTESIAN_POINT('Ctrl Pts',(0.00951081625659959,-0.437096538963801,
-0.245312733520535));
#64722=CARTESIAN_POINT('Ctrl Pts',(0.0317271789964791,-0.436613131466661,
-0.24449883098311));
#64723=CARTESIAN_POINT('Ctrl Pts',(0.053970050068627,-0.434430233866494,
-0.243684928445685));
#64724=CARTESIAN_POINT('Ctrl Pts',(0.0759588056466642,-0.430550925959674,
-0.24287102590826));
#64725=CARTESIAN_POINT('Ctrl Pts',(0.0979083516421918,-0.426678535499496,
-0.242058574693471));
#64726=CARTESIAN_POINT('Ctrl Pts',(0.119603975224661,-0.421115807505287,
-0.241246123478681));
#64727=CARTESIAN_POINT('Ctrl Pts',(0.140769515543163,-0.413917604715894,
-0.240433672263892));
#64728=CARTESIAN_POINT('Ctrl Pts',(0.161912624805773,-0.40672703051933,
-0.239622082077847));
#64729=CARTESIAN_POINT('Ctrl Pts',(0.182526083246665,-0.39790462540619,
-0.238810491891802));
#64730=CARTESIAN_POINT('Ctrl Pts',(0.202348109039612,-0.387555264147054,
-0.237998901705757));
#64731=CARTESIAN_POINT('Ctrl Pts',(0.222179662922132,-0.377200928136997,
-0.237186921402977));
#64732=CARTESIAN_POINT('Ctrl Pts',(0.241218381327371,-0.36531848427911,
-0.236374941100197));
#64733=CARTESIAN_POINT('Ctrl Pts',(0.259225658378425,-0.352059509228585,
-0.235562960797416));
#64734=CARTESIAN_POINT('Ctrl Pts',(0.277237364648469,-0.338797272890752,
-0.234750780773237));
#64735=CARTESIAN_POINT('Ctrl Pts',(0.294216567259407,-0.32415828071142,
-0.233938600749057));
#64736=CARTESIAN_POINT('Ctrl Pts',(0.309957052119384,-0.308334989648371,
-0.233126420724877));
#64737=CARTESIAN_POINT('Ctrl Pts',(0.325731348562761,-0.292477709128823,
-0.232312496085276));
#64738=CARTESIAN_POINT('Ctrl Pts',(0.340261144854378,-0.275431591742576,
-0.231498571445675));
#64739=CARTESIAN_POINT('Ctrl Pts',(0.353379229979316,-0.25742369708173,
-0.230684646806073));
#64740=CARTESIAN_POINT('Ctrl Pts',(0.359794272983742,-0.248617425619982,
-0.230286619082082));
#64741=CARTESIAN_POINT('Ctrl Pts',(0.365872369471393,-0.239581604847051,
-0.229888591358091));
#64742=CARTESIAN_POINT('Ctrl Pts',(0.371597910291157,-0.230345030480897,
-0.2294905636341));
#64743=CARTESIAN_POINT('Ctrl Pts',(0.383302953098264,-0.211462185741816,
-0.228676853332419));
#64744=CARTESIAN_POINT('Ctrl Pts',(0.393598548054935,-0.191630784443394,
-0.227863143030739));
#64745=CARTESIAN_POINT('Ctrl Pts',(0.402334272718512,-0.171087617892312,
-0.227049432729058));
#64746=CARTESIAN_POINT('Ctrl Pts',(0.411054413010577,-0.150581099971071,
-0.226237174071532));
#64747=CARTESIAN_POINT('Ctrl Pts',(0.418219878496133,-0.129365966855261,
-0.225424915414007));
#64748=CARTESIAN_POINT('Ctrl Pts',(0.42372608260923,-0.107703513947485,
-0.224612656756481));
#64749=CARTESIAN_POINT('Ctrl Pts',(0.429226451898634,-0.0860640163444657,
-0.223801258834584));
#64750=CARTESIAN_POINT('Ctrl Pts',(0.433070848035163,-0.0639788233525656,
-0.222989860912687));
#64751=CARTESIAN_POINT('Ctrl Pts',(0.435204446264768,-0.0417244526791764,
-0.22217846299079));
#64752=CARTESIAN_POINT('Ctrl Pts',(0.437339077286187,-0.0194593095315962,
-0.221366672302758));
#64753=CARTESIAN_POINT('Ctrl Pts',(0.437761169140678,0.00297446411620671,
-0.220554881614725));
#64754=CARTESIAN_POINT('Ctrl Pts',(0.436467682495792,0.0252943103632527,
-0.219743090926692));
#64755=CARTESIAN_POINT('Ctrl Pts',(0.435173875617286,0.0476196824231763,
-0.218931099260419));
#64756=CARTESIAN_POINT('Ctrl Pts',(0.4321637176653,0.0698303584049589,-0.218119107594145));
#64757=CARTESIAN_POINT('Ctrl Pts',(0.427486099801381,0.0916486468891051,
-0.217307115927871));
#64758=CARTESIAN_POINT('Ctrl Pts',(0.422798403889784,0.113513943435468,
-0.216493374804724));
#64759=CARTESIAN_POINT('Ctrl Pts',(0.416436272878416,0.13498447528246,-0.215679633681576));
#64760=CARTESIAN_POINT('Ctrl Pts',(0.40849886971943,0.155796384547101,-0.214865892558429));
#64761=CARTESIAN_POINT('Ctrl Pts',(0.40460531742823,0.166005297384021,-0.214466726288175));
#64762=CARTESIAN_POINT('Ctrl Pts',(0.400333460376828,0.17605603414868,-0.21406756001792));
#64763=CARTESIAN_POINT('Ctrl Pts',(0.395699074473075,0.185919559114021,
-0.213668393747666));
#64764=CARTESIAN_POINT('Ctrl Pts',(0.386248884447322,0.206032727758595,
-0.212854435397172));
#64765=CARTESIAN_POINT('Ctrl Pts',(0.375234272621707,0.225481003321121,
-0.212040477046679));
#64766=CARTESIAN_POINT('Ctrl Pts',(0.362771836476794,0.244009087247287,
-0.211226518696185));
#64767=CARTESIAN_POINT('Ctrl Pts',(0.350331649792709,0.262504092578487,
-0.210414013523402));
#64768=CARTESIAN_POINT('Ctrl Pts',(0.33644911834653,0.280081549310864,-0.209601508350619));
#64769=CARTESIAN_POINT('Ctrl Pts',(0.321286366746358,0.296511231731489,
-0.208789003177837));
#64770=CARTESIAN_POINT('Ctrl Pts',(0.306139720582353,0.312923463018676,
-0.207977361024547));
#64771=CARTESIAN_POINT('Ctrl Pts',(0.289716016086182,0.328189798415627,
-0.207165718871257));
#64772=CARTESIAN_POINT('Ctrl Pts',(0.272217266964286,0.342113430847861,
-0.206354076717967));
#64773=CARTESIAN_POINT('Ctrl Pts',(0.254710182870472,0.356043695359024,
-0.205542047964783));
#64774=CARTESIAN_POINT('Ctrl Pts',(0.236127579275898,0.368629519174213,
-0.204730019211599));
#64775=CARTESIAN_POINT('Ctrl Pts',(0.216704766697847,0.379714213706087,
-0.203917990458415));
#64776=CARTESIAN_POINT('Ctrl Pts',(0.197277223403594,0.390801608080931,
-0.203105763923496));
#64777=CARTESIAN_POINT('Ctrl Pts',(0.177009700324741,0.40038681807714,-0.202293537388577));
#64778=CARTESIAN_POINT('Ctrl Pts',(0.156161749713277,0.408359336769086,
-0.201481310853657));
#64779=CARTESIAN_POINT('Ctrl Pts',(0.135269112674117,0.416348944113376,
-0.200667343356137));
#64780=CARTESIAN_POINT('Ctrl Pts',(0.113794249235171,0.422718748466058,
-0.199853375858616));
#64781=CARTESIAN_POINT('Ctrl Pts',(0.0920125345055164,0.427407923995182,
-0.199039408361096));
#64782=CARTESIAN_POINT('Ctrl Pts',(0.0813693558875901,0.429699191388346,
-0.198641680194474));
#64783=CARTESIAN_POINT('Ctrl Pts',(0.0706530627684541,0.431589976052635,
-0.198243952027853));
#64784=CARTESIAN_POINT('Ctrl Pts',(0.0598962310386143,0.433077685302959,
-0.197846223861231));
#64785=CARTESIAN_POINT('Ctrl Pts',(0.0370685737600804,0.436234833964334,
-0.197002183301178));
#64786=CARTESIAN_POINT('Ctrl Pts',(0.0139233262192277,0.437591464740278,
-0.196158142741124));
#64787=CARTESIAN_POINT('Ctrl Pts',(-0.00922985932074797,0.43710256198851,
-0.195314102181071));
#64788=CARTESIAN_POINT('Origin',(0.,0.,-0.425));
#64789=CARTESIAN_POINT('',(-0.494199919830197,0.000281495695726044,-0.703567954531148));
#64790=CARTESIAN_POINT('',(0.217103634412858,0.443959065595836,-0.735793298822188));
#64791=CARTESIAN_POINT('Ctrl Pts',(-0.494199919830141,0.000281495793510342,
-0.70356795453431));
#64792=CARTESIAN_POINT('Ctrl Pts',(-0.494189043315793,0.0193765325329848,
-0.704185398288897));
#64793=CARTESIAN_POINT('Ctrl Pts',(-0.493071481655549,0.0384371587244305,
-0.704802842043484));
#64794=CARTESIAN_POINT('Ctrl Pts',(-0.490859027051234,0.0573677223037112,
-0.705420285798071));
#64795=CARTESIAN_POINT('Ctrl Pts',(-0.488025007900596,0.0816166174500458,
-0.706211193517275));
#64796=CARTESIAN_POINT('Ctrl Pts',(-0.483382241576563,0.105719856305908,
-0.707002101236479));
#64797=CARTESIAN_POINT('Ctrl Pts',(-0.476961436613325,0.129388670229479,
-0.707793008955683));
#64798=CARTESIAN_POINT('Ctrl Pts',(-0.470551610652628,0.153017012596962,
-0.708582564293386));
#64799=CARTESIAN_POINT('Ctrl Pts',(-0.462369911821056,0.176211732126128,
-0.709372119631088));
#64800=CARTESIAN_POINT('Ctrl Pts',(-0.452498206008631,0.198693265006569,
-0.71016167496879));
#64801=CARTESIAN_POINT('Ctrl Pts',(-0.442636742276802,0.221151472873474,
-0.710950411127968));
#64802=CARTESIAN_POINT('Ctrl Pts',(-0.431089005319465,0.242897323630535,
-0.711739147287145));
#64803=CARTESIAN_POINT('Ctrl Pts',(-0.417985469180945,0.263669845741953,
-0.712527883446322));
#64804=CARTESIAN_POINT('Ctrl Pts',(-0.404876010945428,0.284451755921562,
-0.713316976072028));
#64805=CARTESIAN_POINT('Ctrl Pts',(-0.390209699265885,0.304258863184272,
-0.714106068697735));
#64806=CARTESIAN_POINT('Ctrl Pts',(-0.374161764982923,0.322856955360828,
-0.714895161323441));
#64807=CARTESIAN_POINT('Ctrl Pts',(-0.358110975600725,0.341458356336999,
-0.715684394337169));
#64808=CARTESIAN_POINT('Ctrl Pts',(-0.340678545179392,0.358849808020938,
-0.716473627350897));
#64809=CARTESIAN_POINT('Ctrl Pts',(-0.322078167210184,0.374832354802155,
-0.717262860364625));
#64810=CARTESIAN_POINT('Ctrl Pts',(-0.303437753289581,0.39084930284485,
-0.718053792144616));
#64811=CARTESIAN_POINT('Ctrl Pts',(-0.283624920583873,0.405450867811287,
-0.718844723924608));
#64812=CARTESIAN_POINT('Ctrl Pts',(-0.262885493554465,0.418479219649704,
-0.719635655704599));
#64813=CARTESIAN_POINT('Ctrl Pts',(-0.248841251991481,0.427301706410154,
-0.720171255697901));
#64814=CARTESIAN_POINT('Ctrl Pts',(-0.234372743655487,0.435403667645454,
-0.720706855691203));
#64815=CARTESIAN_POINT('Ctrl Pts',(-0.219562184950262,0.442748333638724,
-0.721242455684505));
#64816=CARTESIAN_POINT('Ctrl Pts',(-0.198162636941886,0.453360528334189,
-0.722016335859998));
#64817=CARTESIAN_POINT('Ctrl Pts',(-0.175919859251839,0.462453061988652,
-0.722790216035492));
#64818=CARTESIAN_POINT('Ctrl Pts',(-0.153080630572819,0.469893562994247,
-0.723564096210985));
#64819=CARTESIAN_POINT('Ctrl Pts',(-0.130281663118874,0.477320947808841,
-0.724336612182618));
#64820=CARTESIAN_POINT('Ctrl Pts',(-0.106888989111418,0.483101796651286,
-0.725109128154251));
#64821=CARTESIAN_POINT('Ctrl Pts',(-0.0831705534104316,0.487151207578717,
-0.725881644125885));
#64822=CARTESIAN_POINT('Ctrl Pts',(-0.0594763804315271,0.491196476170071,
-0.726653369853989));
#64823=CARTESIAN_POINT('Ctrl Pts',(-0.0354578103524282,0.493513670289717,
-0.727425095582093));
#64824=CARTESIAN_POINT('Ctrl Pts',(-0.0113943297299146,0.494068628077118,
-0.728196821310198));
#64825=CARTESIAN_POINT('Ctrl Pts',(0.0126807155116891,0.494623852570552,
-0.728968917920397));
#64826=CARTESIAN_POINT('Ctrl Pts',(0.0367999923064215,0.49341511688943,
-0.729741014530596));
#64827=CARTESIAN_POINT('Ctrl Pts',(0.0606819164688182,0.490460339898825,
-0.730513111140794));
#64828=CARTESIAN_POINT('Ctrl Pts',(0.0845712378333966,0.487504647693741,
-0.731285446900682));
#64829=CARTESIAN_POINT('Ctrl Pts',(0.108222349062157,0.482801966413205,
-0.732057782660569));
#64830=CARTESIAN_POINT('Ctrl Pts',(0.131362496978341,0.476421593116449,
-0.732830118420457));
#64831=CARTESIAN_POINT('Ctrl Pts',(0.15454926048216,0.470028366623956,-0.733604010042711));
#64832=CARTESIAN_POINT('Ctrl Pts',(0.177222330691234,0.461950958188405,
-0.734377901664965));
#64833=CARTESIAN_POINT('Ctrl Pts',(0.199126837746785,0.452307575095715,
-0.735151793287219));
#64834=CARTESIAN_POINT('Ctrl Pts',(0.205179305608705,0.449642997157454,
-0.735365628465542));
#64835=CARTESIAN_POINT('Ctrl Pts',(0.211173242086841,0.44685912964959,-0.735579463643865));
#64836=CARTESIAN_POINT('Ctrl Pts',(0.217103634412858,0.443959065595836,
-0.735793298822188));
#64837=CARTESIAN_POINT('',(-0.21691713542861,0.4440502182833,-0.7358));
#64838=CARTESIAN_POINT('Origin',(0.,0.,-0.7358));
#64839=CARTESIAN_POINT('',(-0.494199978279375,0.000146521891872193,-0.71803204546284));
#64840=CARTESIAN_POINT('Ctrl Pts',(-0.21691713542861,0.444050218283299,
-0.7358));
#64841=CARTESIAN_POINT('Ctrl Pts',(-0.242422499554944,0.431590928102705,
-0.734885845562297));
#64842=CARTESIAN_POINT('Ctrl Pts',(-0.266820316362194,0.416946027148979,
-0.733971691124595));
#64843=CARTESIAN_POINT('Ctrl Pts',(-0.289781003824319,0.400325629734807,
-0.733057536686892));
#64844=CARTESIAN_POINT('Ctrl Pts',(-0.312720563515027,0.383720525937519,
-0.732144223428097));
#64845=CARTESIAN_POINT('Ctrl Pts',(-0.334225451338591,0.365143726777976,
-0.731230910169302));
#64846=CARTESIAN_POINT('Ctrl Pts',(-0.353998238105765,0.344846179358297,
-0.730317596910507));
#64847=CARTESIAN_POINT('Ctrl Pts',(-0.371524830782327,0.326854438985688,
-0.729508036292599));
#64848=CARTESIAN_POINT('Ctrl Pts',(-0.387690835626447,0.307511334928945,
-0.72869847567469));
#64849=CARTESIAN_POINT('Ctrl Pts',(-0.402311589169874,0.287017465007986,
-0.727888915056782));
#64850=CARTESIAN_POINT('Ctrl Pts',(-0.416625437140234,0.266953783782416,
-0.727096347999748));
#64851=CARTESIAN_POINT('Ctrl Pts',(-0.429443326069453,0.24580492972889,
-0.726303780942715));
#64852=CARTESIAN_POINT('Ctrl Pts',(-0.440610621559015,0.223821179000958,
-0.725511213885681));
#64853=CARTESIAN_POINT('Ctrl Pts',(-0.451776489915784,0.20184023770272,
-0.724718748115341));
#64854=CARTESIAN_POINT('Ctrl Pts',(-0.461291885577421,0.179025226576472,
-0.723926282345001));
#64855=CARTESIAN_POINT('Ctrl Pts',(-0.469048899800802,0.155649508819196,
-0.723133816574661));
#64856=CARTESIAN_POINT('Ctrl Pts',(-0.476815701348878,0.132244297015232,
-0.722340350919625));
#64857=CARTESIAN_POINT('Ctrl Pts',(-0.482819504926692,0.108277624151794,
-0.72154688526459));
#64858=CARTESIAN_POINT('Ctrl Pts',(-0.487002394070417,0.0840375402405484,
-0.720753419609555));
#64859=CARTESIAN_POINT('Ctrl Pts',(-0.488365278047467,0.0761395489647055,
-0.720494889777558));
#64860=CARTESIAN_POINT('Ctrl Pts',(-0.489535259913778,0.068212597425999,
-0.720236359945562));
#64861=CARTESIAN_POINT('Ctrl Pts',(-0.490511524358925,0.0602667775070422,
-0.719977830113566));
#64862=CARTESIAN_POINT('Ctrl Pts',(-0.492960758624551,0.0403324507877492,
-0.71932923523094));
#64863=CARTESIAN_POINT('Ctrl Pts',(-0.494194016840838,0.020253694832792,
-0.718680640348315));
#64864=CARTESIAN_POINT('Ctrl Pts',(-0.494199978279349,0.000146521980200406,
-0.718032045465689));
#64865=CARTESIAN_POINT('',(-0.493957328857296,0.000144449760132726,-0.618032048526421));
#64866=CARTESIAN_POINT('Ctrl Pts',(-0.494199978279375,0.000146521891871864,
-0.71803204546284));
#64867=CARTESIAN_POINT('Ctrl Pts',(-0.494207244096923,-0.0243601700993693,
-0.717241535770997));
#64868=CARTESIAN_POINT('Ctrl Pts',(-0.492387304238366,-0.0489116703554373,
-0.716451026079155));
#64869=CARTESIAN_POINT('Ctrl Pts',(-0.488746376918454,-0.0732162485318961,
-0.715660516387312));
#64870=CARTESIAN_POINT('Ctrl Pts',(-0.485109097541938,-0.0974964752951923,
-0.714870798728475));
#64871=CARTESIAN_POINT('Ctrl Pts',(-0.479654529871509,-0.121529589269361,
-0.714081081069639));
#64872=CARTESIAN_POINT('Ctrl Pts',(-0.472440669219862,-0.145029149025596,
-0.713291363410802));
#64873=CARTESIAN_POINT('Ctrl Pts',(-0.46522265817095,-0.168542228936054,
-0.71250119139858));
#64874=CARTESIAN_POINT('Ctrl Pts',(-0.456243513596847,-0.191520475939915,
-0.711711019386358));
#64875=CARTESIAN_POINT('Ctrl Pts',(-0.4456114552376,-0.213691532263279,
-0.710920847374135));
#64876=CARTESIAN_POINT('Ctrl Pts',(-0.43497729975056,-0.235866961732167,
-0.710130519503881));
#64877=CARTESIAN_POINT('Ctrl Pts',(-0.422689903369407,-0.257234273154619,
-0.709340191633627));
#64878=CARTESIAN_POINT('Ctrl Pts',(-0.408903840618506,-0.277545111878116,
-0.708549863763373));
#64879=CARTESIAN_POINT('Ctrl Pts',(-0.395084683632739,-0.297904707935681,
-0.707757638665707));
#64880=CARTESIAN_POINT('Ctrl Pts',(-0.379760090875259,-0.317202212976357,
-0.706965413568041));
#64881=CARTESIAN_POINT('Ctrl Pts',(-0.363126562901895,-0.335220433916336,
-0.706173188470374));
#64882=CARTESIAN_POINT('Ctrl Pts',(-0.349006580853906,-0.350515863521925,
-0.70550067905596));
#64883=CARTESIAN_POINT('Ctrl Pts',(-0.33394424513909,-0.364889857227316,
-0.704828169641546));
#64884=CARTESIAN_POINT('Ctrl Pts',(-0.318078815963211,-0.378232080653455,
-0.704155660227131));
#64885=CARTESIAN_POINT('Ctrl Pts',(-0.299623197393985,-0.393752554993512,
-0.703373356950046));
#64886=CARTESIAN_POINT('Ctrl Pts',(-0.279968336043869,-0.407969816740406,
-0.702591053672961));
#64887=CARTESIAN_POINT('Ctrl Pts',(-0.259326300085853,-0.420694081351024,
-0.701808750395877));
#64888=CARTESIAN_POINT('Ctrl Pts',(-0.238723919473107,-0.433393901420054,
-0.701027949998964));
#64889=CARTESIAN_POINT('Ctrl Pts',(-0.217138687657615,-0.444605994987196,
-0.700247149602051));
#64890=CARTESIAN_POINT('Ctrl Pts',(-0.194814530887546,-0.454181614065415,
-0.699466349205139));
#64891=CARTESIAN_POINT('Ctrl Pts',(-0.172517371391529,-0.463745653059551,
-0.698686493053625));
#64892=CARTESIAN_POINT('Ctrl Pts',(-0.149483692726507,-0.471676835437457,
-0.69790663690211));
#64893=CARTESIAN_POINT('Ctrl Pts',(-0.125980905571912,-0.477872840231877,
-0.697126780750596));
#64894=CARTESIAN_POINT('Ctrl Pts',(-0.102470164077595,-0.484070942017038,
-0.696346660662693));
#64895=CARTESIAN_POINT('Ctrl Pts',(-0.0784906736443169,-0.488532484068602,
-0.69556654057479));
#64896=CARTESIAN_POINT('Ctrl Pts',(-0.0543247696931755,-0.491205109295275,
-0.694786420486887));
#64897=CARTESIAN_POINT('Ctrl Pts',(-0.0301566133277679,-0.493877983627432,
-0.694006227686884));
#64898=CARTESIAN_POINT('Ctrl Pts',(-0.00580271548859992,-0.494761555682616,
-0.693226034886882));
#64899=CARTESIAN_POINT('Ctrl Pts',(0.0184502740422664,-0.493855472165456,
-0.692445842086879));
#64900=CARTESIAN_POINT('Ctrl Pts',(0.0427572233526025,-0.492947372729115,
-0.691663913458335));
#64901=CARTESIAN_POINT('Ctrl Pts',(0.0669621087722994,-0.490241731562058,
-0.690881984829792));
#64902=CARTESIAN_POINT('Ctrl Pts',(0.0907827585528636,-0.485790212694258,
-0.690100056201248));
#64903=CARTESIAN_POINT('Ctrl Pts',(0.108721627968127,-0.482437860159601,
-0.689511200914398));
#64904=CARTESIAN_POINT('Ctrl Pts',(0.126442657763115,-0.478096476634594,
-0.688922345627547));
#64905=CARTESIAN_POINT('Ctrl Pts',(0.143831307851241,-0.472806720427916,
-0.688333490340696));
#64906=CARTESIAN_POINT('Ctrl Pts',(0.16718711327821,-0.46570171135055,-0.687542561232651));
#64907=CARTESIAN_POINT('Ctrl Pts',(0.190077963261476,-0.45684287391047,
-0.686751632124605));
#64908=CARTESIAN_POINT('Ctrl Pts',(0.212225147621608,-0.446311692337302,
-0.685960703016559));
#64909=CARTESIAN_POINT('Ctrl Pts',(0.234334212618236,-0.435798636857817,
-0.685171135242473));
#64910=CARTESIAN_POINT('Ctrl Pts',(0.25570151426798,-0.423619198931231,
-0.684381567468386));
#64911=CARTESIAN_POINT('Ctrl Pts',(0.276066477637526,-0.409903573935151,
-0.6835919996943));
#64912=CARTESIAN_POINT('Ctrl Pts',(0.296410082892266,-0.396202333442886,
-0.682803259993354));
#64913=CARTESIAN_POINT('Ctrl Pts',(0.315752852412834,-0.380968466591575,
-0.682014520292407));
#64914=CARTESIAN_POINT('Ctrl Pts',(0.333861132976999,-0.364376706016335,
-0.681225780591461));
#64915=CARTESIAN_POINT('Ctrl Pts',(0.351977287474953,-0.347777730928168,
-0.680436697926744));
#64916=CARTESIAN_POINT('Ctrl Pts',(0.368857356774819,-0.329820133027349,
-0.679647615262028));
#64917=CARTESIAN_POINT('Ctrl Pts',(0.384301967368983,-0.310717939418259,
-0.678858532597311));
#64918=CARTESIAN_POINT('Ctrl Pts',(0.399749177407836,-0.291612530765616,
-0.678069317124018));
#64919=CARTESIAN_POINT('Ctrl Pts',(0.413760033322562,-0.271362696072906,
-0.677280101650725));
#64920=CARTESIAN_POINT('Ctrl Pts',(0.426176682147419,-0.250214059544658,
-0.676490886177432));
#64921=CARTESIAN_POINT('Ctrl Pts',(0.43861987187072,-0.229020217275132,
-0.675699983736261));
#64922=CARTESIAN_POINT('Ctrl Pts',(0.449461731410235,-0.206924351775776,
-0.674909081295089));
#64923=CARTESIAN_POINT('Ctrl Pts',(0.458590583438979,-0.18419640816557,
-0.674118178853917));
#64924=CARTESIAN_POINT('Ctrl Pts',(0.464772876727418,-0.168804460437752,
-0.673582559387366));
#64925=CARTESIAN_POINT('Ctrl Pts',(0.470170522976654,-0.153123089496478,
-0.673046939920814));
#64926=CARTESIAN_POINT('Ctrl Pts',(0.47476192847652,-0.137239758340124,
-0.672511320454262));
#64927=CARTESIAN_POINT('Ctrl Pts',(0.481535664504905,-0.113806957097083,
-0.671721116914586));
#64928=CARTESIAN_POINT('Ctrl Pts',(0.48658864117106,-0.0898083330886664,
-0.670930913374909));
#64929=CARTESIAN_POINT('Ctrl Pts',(0.489837288117429,-0.0655215321078692,
-0.670140709835232));
#64930=CARTESIAN_POINT('Ctrl Pts',(0.493080401942685,-0.0412760965981491,
-0.669351852176459));
#64931=CARTESIAN_POINT('Ctrl Pts',(0.494525145611274,-0.0167441303366198,
-0.668562994517687));
#64932=CARTESIAN_POINT('Ctrl Pts',(0.494138672924038,0.00778536581481629,
-0.667774136858914));
#64933=CARTESIAN_POINT('Ctrl Pts',(0.493752597210261,0.032289665984111,
-0.666986089491693));
#64934=CARTESIAN_POINT('Ctrl Pts',(0.491539024476357,0.0567908121559613,
-0.666198042124471));
#64935=CARTESIAN_POINT('Ctrl Pts',(0.487517124062875,0.0809981095178388,
-0.66540999475725));
#64936=CARTESIAN_POINT('Ctrl Pts',(0.483493290450566,0.105217042552913,
-0.664621568600877));
#64937=CARTESIAN_POINT('Ctrl Pts',(0.477659485504374,0.129141158390872,
-0.663833142444504));
#64938=CARTESIAN_POINT('Ctrl Pts',(0.470086507952698,0.152487097948771,
-0.663044716288131));
#64939=CARTESIAN_POINT('Ctrl Pts',(0.462512070366296,0.175837538494852,
-0.662256138126875));
#64940=CARTESIAN_POINT('Ctrl Pts',(0.453198031838177,0.198608930707294,
-0.661467559965618));
#64941=CARTESIAN_POINT('Ctrl Pts',(0.442264297449436,0.220535555413535,
-0.660678981804362));
#64942=CARTESIAN_POINT('Ctrl Pts',(0.431306593626934,0.242510248671639,
-0.659888674885911));
#64943=CARTESIAN_POINT('Ctrl Pts',(0.418722446922477,0.263635873164357,
-0.659098367967459));
#64944=CARTESIAN_POINT('Ctrl Pts',(0.404677297416772,0.283672213929136,
-0.658308061049007));
#64945=CARTESIAN_POINT('Ctrl Pts',(0.395086998081313,0.297353414363736,
-0.657768424221947));
#64946=CARTESIAN_POINT('Ctrl Pts',(0.384816459366048,0.310527325364656,
-0.657228787394887));
#64947=CARTESIAN_POINT('Ctrl Pts',(0.373928785729749,0.323126760270139,
-0.656689150567828));
#64948=CARTESIAN_POINT('Ctrl Pts',(0.358022972409093,0.341533287343491,
-0.655900794586661));
#64949=CARTESIAN_POINT('Ctrl Pts',(0.340709666072,0.358814795169719,-0.655112438605495));
#64950=CARTESIAN_POINT('Ctrl Pts',(0.322174116471729,0.374749888159638,
-0.654324082624329));
#64951=CARTESIAN_POINT('Ctrl Pts',(0.303671294869083,0.390656844746979,
-0.653537118633864));
#64952=CARTESIAN_POINT('Ctrl Pts',(0.283950999955547,0.405221616003787,
-0.652750154643398));
#64953=CARTESIAN_POINT('Ctrl Pts',(0.263235856531688,0.418258919613232,
-0.651963190652933));
#64954=CARTESIAN_POINT('Ctrl Pts',(0.242543096654239,0.431282135891278,
-0.651177077008741));
#64955=CARTESIAN_POINT('Ctrl Pts',(0.220858192931202,0.442780768411191,
-0.650390963364548));
#64956=CARTESIAN_POINT('Ctrl Pts',(0.198433747993738,0.452612071930431,
-0.649604849720356));
#64957=CARTESIAN_POINT('Ctrl Pts',(0.175999603359157,0.462447627981525,
-0.648818396042586));
#64958=CARTESIAN_POINT('Ctrl Pts',(0.152825906399773,0.470614113568941,
-0.648031942364815));
#64959=CARTESIAN_POINT('Ctrl Pts',(0.129187428819195,0.477015983207151,
-0.647245488687044));
#64960=CARTESIAN_POINT('Ctrl Pts',(0.105545124682946,0.483418889168894,
-0.646458907699519));
#64961=CARTESIAN_POINT('Ctrl Pts',(0.0814385687965266,0.488056453694102,
-0.645672326711994));
#64962=CARTESIAN_POINT('Ctrl Pts',(0.0571546618842482,0.490883880999262,
-0.644885745724469));
#64963=CARTESIAN_POINT('Ctrl Pts',(0.032817603107085,0.493717496889916,
-0.64409744309279));
#64964=CARTESIAN_POINT('Ctrl Pts',(0.0083031147787867,0.494733021134595,
-0.643309140461111));
#64965=CARTESIAN_POINT('Ctrl Pts',(-0.0160983489333721,0.493937732069154,
-0.642520837829432));
#64966=CARTESIAN_POINT('Ctrl Pts',(-0.0331630875930237,0.493381560512369,
-0.641969552113419));
#64967=CARTESIAN_POINT('Ctrl Pts',(-0.0501725070709088,0.49194089521943,
-0.641418266397407));
#64968=CARTESIAN_POINT('Ctrl Pts',(-0.067029536706112,0.489633210892566,
-0.640866980681394));
#64969=CARTESIAN_POINT('Ctrl Pts',(-0.0911731719304014,0.486328008860752,
-0.640077396660969));
#64970=CARTESIAN_POINT('Ctrl Pts',(-0.115138288037024,0.481223649190943,
-0.639287812640545));
#64971=CARTESIAN_POINT('Ctrl Pts',(-0.138637569592122,0.474355630616513,
-0.638498228620121));
#64972=CARTESIAN_POINT('Ctrl Pts',(-0.162096057117822,0.467499534710909,
-0.63771001529325));
#64973=CARTESIAN_POINT('Ctrl Pts',(-0.185089642614131,0.458885999687149,
-0.63692180196638));
#64974=CARTESIAN_POINT('Ctrl Pts',(-0.207341068124737,0.448601517461648,
-0.636133588639509));
#64975=CARTESIAN_POINT('Ctrl Pts',(-0.229568978728543,0.438327903692233,
-0.635346208282324));
#64976=CARTESIAN_POINT('Ctrl Pts',(-0.25105564894622,0.426387113204784,
-0.63455882792514));
#64977=CARTESIAN_POINT('Ctrl Pts',(-0.271543256460522,0.412913913389723,
-0.633771447567955));
#64978=CARTESIAN_POINT('Ctrl Pts',(-0.292040020441645,0.399434692036666,
-0.632983715309158));
#64979=CARTESIAN_POINT('Ctrl Pts',(-0.3115362382033,0.384422055600117,-0.632195983050361));
#64980=CARTESIAN_POINT('Ctrl Pts',(-0.329801650634823,0.368055038327892,
-0.631408250791564));
#64981=CARTESIAN_POINT('Ctrl Pts',(-0.348070214991009,0.351685196722759,
-0.630620382599744));
#64982=CARTESIAN_POINT('Ctrl Pts',(-0.365107052144935,0.333960991305438,
-0.629832514407923));
#64983=CARTESIAN_POINT('Ctrl Pts',(-0.380717878936952,0.315099248900642,
-0.629044646216103));
#64984=CARTESIAN_POINT('Ctrl Pts',(-0.396362675980733,0.296196462024162,
-0.628255063567951));
#64985=CARTESIAN_POINT('Ctrl Pts',(-0.410574852499632,0.27615175415103,
-0.627465480919799));
#64986=CARTESIAN_POINT('Ctrl Pts',(-0.423201864383091,0.255213287237706,
-0.626675898271647));
#64987=CARTESIAN_POINT('Ctrl Pts',(-0.431896652276968,0.240795344947433,
-0.626132202446085));
#64988=CARTESIAN_POINT('Ctrl Pts',(-0.439840744309758,0.22595425813607,
-0.625588506620522));
#64989=CARTESIAN_POINT('Ctrl Pts',(-0.446997421954708,0.210777002459577,
-0.625044810794959));
#64990=CARTESIAN_POINT('Ctrl Pts',(-0.458220859400495,0.186975318475107,
-0.624192161508451));
#64991=CARTESIAN_POINT('Ctrl Pts',(-0.467560202617464,0.162231059761754,
-0.623339512221943));
#64992=CARTESIAN_POINT('Ctrl Pts',(-0.474875071827669,0.13684774808767,
-0.622486862935434));
#64993=CARTESIAN_POINT('Ctrl Pts',(-0.482151827518084,0.111596694055384,
-0.621638656307369));
#64994=CARTESIAN_POINT('Ctrl Pts',(-0.487424918762182,0.0857136895848494,
-0.620790449679303));
#64995=CARTESIAN_POINT('Ctrl Pts',(-0.490602792428975,0.0595192410980851,
-0.619942243051237));
#64996=CARTESIAN_POINT('Ctrl Pts',(-0.492988355924927,0.0398556148313835,
-0.619305512022537));
#64997=CARTESIAN_POINT('Ctrl Pts',(-0.49419416568895,0.020016978509648,
-0.618668780993836));
#64998=CARTESIAN_POINT('Ctrl Pts',(-0.494199978855518,0.000144565574625915,
-0.618032049965136));
#64999=CARTESIAN_POINT('',(-0.494183370864054,-0.00044364358185519,-0.518032045465689));
#65000=CARTESIAN_POINT('Ctrl Pts',(-0.493441113705293,0.000144203375642127,
-0.618032045465689));
#65001=CARTESIAN_POINT('Ctrl Pts',(-0.49319563664091,-0.0913624936415018,
-0.615095577279967));
#65002=CARTESIAN_POINT('Ctrl Pts',(-0.42500180876295,-0.347559668173545,
-0.606885052465435));
#65003=CARTESIAN_POINT('Ctrl Pts',(-0.0134997172395283,-0.583292780708831,
-0.59340047102209));
#65004=CARTESIAN_POINT('Ctrl Pts',(0.481597770827401,-0.329343127216554,
-0.577578301135657));
#65005=CARTESIAN_POINT('Ctrl Pts',(0.538669550813453,0.224150668479914,
-0.561756131249221));
#65006=CARTESIAN_POINT('Ctrl Pts',(0.105791851363253,0.573773597596928,
-0.545933961362787));
#65007=CARTESIAN_POINT('Ctrl Pts',(-0.381589922382086,0.415101937259952,
-0.531359266101609));
#65008=CARTESIAN_POINT('Ctrl Pts',(-0.493051107525581,0.124562909647714,
-0.522058627469244));
#65009=CARTESIAN_POINT('Ctrl Pts',(-0.494183370864054,-0.00044364358185519,
-0.518032045465689));
#65010=CARTESIAN_POINT('',(-0.494856786895912,0.000236248404645519,-0.418032045465689));
#65011=CARTESIAN_POINT('Ctrl Pts',(-0.494183370864054,-0.00044364358185519,
-0.518032045465689));
#65012=CARTESIAN_POINT('Ctrl Pts',(-0.49453415715938,-0.0391719007009277,
-0.516784570840433));
#65013=CARTESIAN_POINT('Ctrl Pts',(-0.472722741173915,-0.241244450658913,
-0.510263039586364));
#65014=CARTESIAN_POINT('Ctrl Pts',(-0.195405102640593,-0.549749372943316,
-0.498467451703485));
#65015=CARTESIAN_POINT('Ctrl Pts',(0.354308135899791,-0.463544097374131,
-0.482645281817051));
#65016=CARTESIAN_POINT('Ctrl Pts',(0.581762127488868,0.0442755404655635,
-0.466823111930615));
#65017=CARTESIAN_POINT('Ctrl Pts',(0.280076793883528,0.511824640016281,
-0.451000942044181));
#65018=CARTESIAN_POINT('Ctrl Pts',(-0.276351126568424,0.513845803011739,
-0.435178772157748));
#65019=CARTESIAN_POINT('Ctrl Pts',(-0.488246889901193,0.190630286924777,
-0.424189139964916));
#65020=CARTESIAN_POINT('Ctrl Pts',(-0.494937727816466,0.0138949803393536,
-0.418473564400897));
#65021=CARTESIAN_POINT('Ctrl Pts',(-0.494856786895912,0.000236248404645519,
-0.418032045465689));
#65022=CARTESIAN_POINT('',(-0.493522771508053,0.000241867023412317,-0.318032045465689));
#65023=CARTESIAN_POINT('Ctrl Pts',(-0.494856786895912,0.000236248404645519,
-0.418032045465689));
#65024=CARTESIAN_POINT('Ctrl Pts',(-0.493970867814446,-0.149262066747403,
-0.413199507772085));
#65025=CARTESIAN_POINT('Ctrl Pts',(-0.34234445800717,-0.463474892665707,
-0.403092913449672));
#65026=CARTESIAN_POINT('Ctrl Pts',(0.191406249927459,-0.551154335841721,
-0.387712262498443));
#65027=CARTESIAN_POINT('Ctrl Pts',(0.566386150012029,-0.140050711081548,
-0.37189009261201));
#65028=CARTESIAN_POINT('Ctrl Pts',(0.426211974611545,0.398435501884038,
-0.356067922725576));
#65029=CARTESIAN_POINT('Ctrl Pts',(-0.101621460572443,0.574526295417654,
-0.34024575283914));
#65030=CARTESIAN_POINT('Ctrl Pts',(-0.450519577851589,0.296895367549325,
-0.327567127085845));
#65031=CARTESIAN_POINT('Ctrl Pts',(-0.493818787931586,0.0666086579641146,
-0.320162557961362));
#65032=CARTESIAN_POINT('Ctrl Pts',(-0.493522771508053,0.000241867023412317,
-0.318032045465689));
#65033=CARTESIAN_POINT('',(-0.494175246121693,-0.000437982247251857,-0.218032043771887));
#65034=CARTESIAN_POINT('Ctrl Pts',(-0.493522771508053,0.000241867023412317,
-0.318032045465689));
#65035=CARTESIAN_POINT('Ctrl Pts',(-0.493086003034083,-0.0976814902536105,
-0.31488850133255));
#65036=CARTESIAN_POINT('Ctrl Pts',(-0.417562805783599,-0.360516000773604,
-0.3064709005706));
#65037=CARTESIAN_POINT('Ctrl Pts',(0.00926706993024401,-0.583370379414318,
-0.292779243179837));
#65038=CARTESIAN_POINT('Ctrl Pts',(0.49408565294531,-0.310302150601255,
-0.276957073293404));
#65039=CARTESIAN_POINT('Ctrl Pts',(0.529510809583032,0.245003489134929,
-0.26113490340697));
#65040=CARTESIAN_POINT('Ctrl Pts',(0.0833216145626671,0.577460662606022,
-0.245312733520534));
#65041=CARTESIAN_POINT('Ctrl Pts',(-0.390666567691133,0.402424062808438,
-0.230945114206776));
#65042=CARTESIAN_POINT('Ctrl Pts',(-0.492979328796984,0.118255994136513,
-0.221851551521826));
#65043=CARTESIAN_POINT('Ctrl Pts',(-0.493995525633567,-0.000437770324621543,
-0.218032045465689));
#65044=CARTESIAN_POINT('',(-0.490426859062112,0.0609519147399937,-0.120013405629935));
#65045=CARTESIAN_POINT('Ctrl Pts',(-0.494199805894521,-0.000438011207620882,
-0.21803204354042));
#65046=CARTESIAN_POINT('Ctrl Pts',(-0.494172750277752,-0.0309643546498033,
-0.217050118877898));
#65047=CARTESIAN_POINT('Ctrl Pts',(-0.491313369343038,-0.0613653915007896,
-0.216068194215376));
#65048=CARTESIAN_POINT('Ctrl Pts',(-0.485713819065904,-0.0911906024128288,
-0.215086269552854));
#65049=CARTESIAN_POINT('Ctrl Pts',(-0.483018613360579,-0.105546233603582,
-0.214613644284458));
#65050=CARTESIAN_POINT('Ctrl Pts',(-0.479689296480285,-0.11976880665172,
-0.214141019016061));
#65051=CARTESIAN_POINT('Ctrl Pts',(-0.475740012640402,-0.133809866500606,
-0.213668393747665));
#65052=CARTESIAN_POINT('Ctrl Pts',(-0.46914374763369,-0.15726185311221,
-0.212878994543758));
#65053=CARTESIAN_POINT('Ctrl Pts',(-0.46079092504738,-0.180289888503342,
-0.21208959533985));
#65054=CARTESIAN_POINT('Ctrl Pts',(-0.450756093102774,-0.202614373948947,
-0.211300196135942));
#65055=CARTESIAN_POINT('Ctrl Pts',(-0.440738742206839,-0.224899969314599,
-0.210512172094666));
#65056=CARTESIAN_POINT('Ctrl Pts',(-0.429045431654185,-0.246483800410652,
-0.20972414805339));
#65057=CARTESIAN_POINT('Ctrl Pts',(-0.415799841100531,-0.267103223755861,
-0.208936124012114));
#65058=CARTESIAN_POINT('Ctrl Pts',(-0.402568315817015,-0.287700751681739,
-0.208148936760333));
#65059=CARTESIAN_POINT('Ctrl Pts',(-0.387788132945832,-0.307335309549207,
-0.207361749508551));
#65060=CARTESIAN_POINT('Ctrl Pts',(-0.3716281231461,-0.325770130746985,
-0.206574562256769));
#65061=CARTESIAN_POINT('Ctrl Pts',(-0.355460960498201,-0.344213111684677,
-0.205787026575069));
#65062=CARTESIAN_POINT('Ctrl Pts',(-0.337913191277882,-0.361454758624169,
-0.204999490893369));
#65063=CARTESIAN_POINT('Ctrl Pts',(-0.319193707533974,-0.377291686988616,
-0.204211955211669));
#65064=CARTESIAN_POINT('Ctrl Pts',(-0.300471045810742,-0.393131303965184,
-0.20342428583119));
#65065=CARTESIAN_POINT('Ctrl Pts',(-0.28057682017882,-0.407565299330699,
-0.202636616450712));
#65066=CARTESIAN_POINT('Ctrl Pts',(-0.259752412171317,-0.420431117272714,
-0.201848947070233));
#65067=CARTESIAN_POINT('Ctrl Pts',(-0.238882683742495,-0.433324935256292,
-0.201059563474966));
#65068=CARTESIAN_POINT('Ctrl Pts',(-0.217079341425805,-0.444643427712769,
-0.200270179879698));
#65069=CARTESIAN_POINT('Ctrl Pts',(-0.194609064591469,-0.454269690799236,
-0.19948079628443));
#65070=CARTESIAN_POINT('Ctrl Pts',(-0.179099370244633,-0.460914041435148,
-0.198935938810031));
#65071=CARTESIAN_POINT('Ctrl Pts',(-0.163272437722091,-0.466753171034724,
-0.198391081335632));
#65072=CARTESIAN_POINT('Ctrl Pts',(-0.147220088809954,-0.471762530783009,
-0.197846223861232));
#65073=CARTESIAN_POINT('Ctrl Pts',(-0.123957690090648,-0.479021887306522,
-0.197056638992124));
#65074=CARTESIAN_POINT('Ctrl Pts',(-0.100092955879836,-0.484576542004863,
-0.196267054123016));
#65075=CARTESIAN_POINT('Ctrl Pts',(-0.0759010851752448,-0.488336631095006,
-0.195477469253907));
#65076=CARTESIAN_POINT('Ctrl Pts',(-0.0517512198782043,-0.492090191377329,
-0.194689255375684));
#65077=CARTESIAN_POINT('Ctrl Pts',(-0.0272760151105899,-0.494055214548706,
-0.19390104149746));
#65078=CARTESIAN_POINT('Ctrl Pts',(-0.00276321768710077,-0.494192274957848,
-0.193112827619237));
#65079=CARTESIAN_POINT('Ctrl Pts',(0.0217236658700617,-0.494329190472671,
-0.192325447006541));
#65080=CARTESIAN_POINT('Ctrl Pts',(0.046247373601404,-0.492641948741059,
-0.191538066393845));
#65081=CARTESIAN_POINT('Ctrl Pts',(0.0705172555593016,-0.489143084044315,
-0.190750685781149));
#65082=CARTESIAN_POINT('Ctrl Pts',(0.0947979704728245,-0.485642657615789,
-0.189962953718073));
#65083=CARTESIAN_POINT('Ctrl Pts',(0.11882394383847,-0.48032906976862,-0.189175221654997));
#65084=CARTESIAN_POINT('Ctrl Pts',(0.142310683354916,-0.473266636689147,
-0.188387489591921));
#65085=CARTESIAN_POINT('Ctrl Pts',(0.165801468263671,-0.466202987165286,
-0.187599621848657));
#65086=CARTESIAN_POINT('Ctrl Pts',(0.1887521778002,-0.45739011747967,-0.186811754105393));
#65087=CARTESIAN_POINT('Ctrl Pts',(0.210894842896268,-0.446941836528825,
-0.186023886362129));
#65088=CARTESIAN_POINT('Ctrl Pts',(0.233085680856849,-0.436470824636584,
-0.185234304559338));
#65089=CARTESIAN_POINT('Ctrl Pts',(0.254464352083612,-0.424357627123245,
-0.184444722756548));
#65090=CARTESIAN_POINT('Ctrl Pts',(0.274787370646444,-0.410762146422007,
-0.183655140953757));
#65091=CARTESIAN_POINT('Ctrl Pts',(0.288781534322225,-0.401400476963514,
-0.183111445294104));
#65092=CARTESIAN_POINT('Ctrl Pts',(0.302275715266755,-0.391336939837268,
-0.18256774963445));
#65093=CARTESIAN_POINT('Ctrl Pts',(0.315199736804966,-0.380634688274834,
-0.182024053974797));
#65094=CARTESIAN_POINT('Ctrl Pts',(0.333938307202834,-0.365117467591981,
-0.181235748309775));
#65095=CARTESIAN_POINT('Ctrl Pts',(0.351580955646325,-0.348169540189685,
-0.180447442644754));
#65096=CARTESIAN_POINT('Ctrl Pts',(0.367902590472904,-0.329971701700808,
-0.179659136979733));
#65097=CARTESIAN_POINT('Ctrl Pts',(0.38419576896201,-0.311805590660732,
-0.178872205704732));
#65098=CARTESIAN_POINT('Ctrl Pts',(0.399172006415922,-0.292394370584428,
-0.178085274429732));
#65099=CARTESIAN_POINT('Ctrl Pts',(0.412641578489278,-0.27195692251141,
-0.177298343154732));
#65100=CARTESIAN_POINT('Ctrl Pts',(0.426096895277571,-0.251541104052655,
-0.176512244714627));
#65101=CARTESIAN_POINT('Ctrl Pts',(0.438048308175922,-0.230101776433988,
-0.175726146274522));
#65102=CARTESIAN_POINT('Ctrl Pts',(0.448348028550459,-0.207888636762371,
-0.174940047834417));
#65103=CARTESIAN_POINT('Ctrl Pts',(0.45865255445566,-0.185665133127465,
-0.174153582625116));
#65104=CARTESIAN_POINT('Ctrl Pts',(0.467303535332435,-0.162667718136668,
-0.173367117415816));
#65105=CARTESIAN_POINT('Ctrl Pts',(0.474199930407406,-0.139169199184342,
-0.172580652206515));
#65106=CARTESIAN_POINT('Ctrl Pts',(0.481097573071553,-0.115666429243265,
-0.171794044722088));
#65107=CARTESIAN_POINT('Ctrl Pts',(0.48623982790186,-0.0916630503429066,
-0.17100743723766));
#65108=CARTESIAN_POINT('Ctrl Pts',(0.489576155418217,-0.0674450001550752,
-0.170220829753233));
#65109=CARTESIAN_POINT('Ctrl Pts',(0.492919884988233,-0.0431732192390262,
-0.169432477083185));
#65110=CARTESIAN_POINT('Ctrl Pts',(0.494449629709502,-0.0186865116197863,
-0.168644124413136));
#65111=CARTESIAN_POINT('Ctrl Pts',(0.494166843308743,0.00572459380850489,
-0.167855771743088));
#65112=CARTESIAN_POINT('Ctrl Pts',(0.493969090469221,0.0227953065491065,
-0.167304475858179));
#65113=CARTESIAN_POINT('Ctrl Pts',(0.492886082646355,0.0398289838668983,
-0.166753179973271));
#65114=CARTESIAN_POINT('Ctrl Pts',(0.490933341258643,0.0567282508158417,
-0.166201884088363));
#65115=CARTESIAN_POINT('Ctrl Pts',(0.488133993899746,0.0809541511826329,
-0.165411575300368));
#65116=CARTESIAN_POINT('Ctrl Pts',(0.483529467227842,0.105038900077909,
-0.164621266512374));
#65117=CARTESIAN_POINT('Ctrl Pts',(0.477149307483064,0.128694127171494,
-0.163830957724379));
#65118=CARTESIAN_POINT('Ctrl Pts',(0.470780310953839,0.152307965270199,
-0.163042031721097));
#65119=CARTESIAN_POINT('Ctrl Pts',(0.462641976466881,0.175493099130243,
-0.162253105717814));
#65120=CARTESIAN_POINT('Ctrl Pts',(0.452815041473334,0.197970144757997,
-0.161464179714532));
#65121=CARTESIAN_POINT('Ctrl Pts',(0.442998656932671,0.220423058445223,
-0.160676100722716));
#65122=CARTESIAN_POINT('Ctrl Pts',(0.43149752188693,0.24216875149014,-0.159888021730901));
#65123=CARTESIAN_POINT('Ctrl Pts',(0.418441051031408,0.262946243197598,
-0.159099942739085));
#65124=CARTESIAN_POINT('Ctrl Pts',(0.405379232005872,0.283732245746872,
-0.158311540935655));
#65125=CARTESIAN_POINT('Ctrl Pts',(0.39076115327825,0.303548656609079,-0.157523139132226));
#65126=CARTESIAN_POINT('Ctrl Pts',(0.374761072967117,0.322161105952496,
-0.156734737328796));
#65127=CARTESIAN_POINT('Ctrl Pts',(0.358758544707163,0.340776402926834,
-0.155946214903018));
#65128=CARTESIAN_POINT('Ctrl Pts',(0.341374064153866,0.358186863061602,
-0.155157692477239));
#65129=CARTESIAN_POINT('Ctrl Pts',(0.322820463086095,0.374193250357191,
-0.154369170051461));
#65130=CARTESIAN_POINT('Ctrl Pts',(0.304227342540955,0.390233731522653,
-0.153578968059864));
#65131=CARTESIAN_POINT('Ctrl Pts',(0.284460677467843,0.40486374277383,-0.152788766068268));
#65132=CARTESIAN_POINT('Ctrl Pts',(0.263765544119174,0.417925086272069,
-0.151998564076671));
#65133=CARTESIAN_POINT('Ctrl Pts',(0.249633160085072,0.42684447418847,-0.151458947451757));
#65134=CARTESIAN_POINT('Ctrl Pts',(0.235068449819283,0.435033240514805,
-0.150919330826843));
#65135=CARTESIAN_POINT('Ctrl Pts',(0.220155539841901,0.442453588839463,
-0.150379714201929));
#65136=CARTESIAN_POINT('Ctrl Pts',(0.198298032359417,0.453329421877741,
-0.149588810586563));
#65137=CARTESIAN_POINT('Ctrl Pts',(0.175574231759261,0.462610811271088,
-0.148797906971198));
#65138=CARTESIAN_POINT('Ctrl Pts',(0.152242765825034,0.470165694467327,
-0.148007003355832));
#65139=CARTESIAN_POINT('Ctrl Pts',(0.128951195010208,0.477707659359674,
-0.14721745212845));
#65140=CARTESIAN_POINT('Ctrl Pts',(0.105054656046012,0.483528720307415,
-0.146427900901068));
#65141=CARTESIAN_POINT('Ctrl Pts',(0.0808320197756471,0.487544689827496,
-0.145638349673686));
#65142=CARTESIAN_POINT('Ctrl Pts',(0.0566345148620286,0.491556492717588,
-0.144849617617816));
#65143=CARTESIAN_POINT('Ctrl Pts',(0.0321122579899425,0.49376678450621,
-0.144060885561945));
#65144=CARTESIAN_POINT('Ctrl Pts',(0.00755510785655334,0.494142247075957,
-0.143272153506075));
#65145=CARTESIAN_POINT('Ctrl Pts',(-0.0170131427268601,0.494517879364236,
-0.142483064923461));
#65146=CARTESIAN_POINT('Ctrl Pts',(-0.0416156278715312,0.493056993651087,
-0.141693976340847));
#65147=CARTESIAN_POINT('Ctrl Pts',(-0.065960445619597,0.48977837805855,
-0.140904887758233));
#65148=CARTESIAN_POINT('Ctrl Pts',(-0.0903095954698473,0.486499179044198,
-0.14011565875919));
#65149=CARTESIAN_POINT('Ctrl Pts',(-0.114400305547835,0.48140172413962,
-0.139326429760147));
#65150=CARTESIAN_POINT('Ctrl Pts',(-0.137949186516829,0.474556279001074,
-0.138537200761103));
#65151=CARTESIAN_POINT('Ctrl Pts',(-0.161548758335482,0.467696098494388,
-0.13774627288352));
#65152=CARTESIAN_POINT('Ctrl Pts',(-0.184603518314131,0.459080642868388,
-0.136955345005936));
#65153=CARTESIAN_POINT('Ctrl Pts',(-0.206846964820815,0.448829559125083,
-0.136164417128352));
#65154=CARTESIAN_POINT('Ctrl Pts',(-0.221910449313245,0.441887422664734,
-0.135628792857399));
#65155=CARTESIAN_POINT('Ctrl Pts',(-0.23660225795376,0.434196191489723,
-0.135093168586447));
#65156=CARTESIAN_POINT('Ctrl Pts',(-0.250846662107074,0.425804640779946,
-0.134557544315494));
#65157=CARTESIAN_POINT('Ctrl Pts',(-0.271427480270615,0.413680231965847,
-0.133783655453187));
#65158=CARTESIAN_POINT('Ctrl Pts',(-0.291196252392501,0.400019231727095,
-0.13300976659088));
#65159=CARTESIAN_POINT('Ctrl Pts',(-0.309907271780441,0.384956001248979,
-0.132235877728573));
#65160=CARTESIAN_POINT('Ctrl Pts',(-0.328585302606954,0.369919328078811,
-0.131463353275106));
#65161=CARTESIAN_POINT('Ctrl Pts',(-0.346208685401953,0.35348572733314,
-0.13069082882164));
#65162=CARTESIAN_POINT('Ctrl Pts',(-0.362559905979217,0.335833224348547,
-0.129918304368173));
#65163=CARTESIAN_POINT('Ctrl Pts',(-0.378894395704946,0.318198783710141,
-0.129146570375081));
#65164=CARTESIAN_POINT('Ctrl Pts',(-0.393958795340787,0.299348422171846,
-0.128374836381989));
#65165=CARTESIAN_POINT('Ctrl Pts',(-0.407571780799048,0.279497555438849,
-0.127603102388897));
#65166=CARTESIAN_POINT('Ctrl Pts',(-0.421191283860761,0.259637184539559,
-0.126830998906235));
#65167=CARTESIAN_POINT('Ctrl Pts',(-0.433357563228689,0.238775938819434,
-0.126058895423573));
#65168=CARTESIAN_POINT('Ctrl Pts',(-0.443931768323362,0.217159446198623,
-0.125286791940911));
#65169=CARTESIAN_POINT('Ctrl Pts',(-0.454509246755392,0.195536262004101,
-0.124514449446886));
#65170=CARTESIAN_POINT('Ctrl Pts',(-0.463493389163292,0.173158031484789,
-0.123742106952861));
#65171=CARTESIAN_POINT('Ctrl Pts',(-0.470793200383583,0.150291059190437,
-0.122969764458837));
#65172=CARTESIAN_POINT('Ctrl Pts',(-0.478107688939874,0.12737810951043,
-0.12219586905749));
#65173=CARTESIAN_POINT('Ctrl Pts',(-0.483730932047285,0.103975162145308,
-0.121421973656143));
#65174=CARTESIAN_POINT('Ctrl Pts',(-0.487622669413537,0.0803602655173329,
-0.120648078254796));
#65175=CARTESIAN_POINT('Ctrl Pts',(-0.488686542371567,0.0739047297077928,
-0.120436520713176));
#65176=CARTESIAN_POINT('Ctrl Pts',(-0.489621320718089,0.0674333787202251,
-0.120224963171555));
#65177=CARTESIAN_POINT('Ctrl Pts',(-0.490426859062112,0.0609519147399937,
-0.120013405629935));
#65178=CARTESIAN_POINT('',(-0.253382212491109,0.424300712223195,-0.12));
#65179=CARTESIAN_POINT('Origin',(0.,0.,-0.12));
#65180=CARTESIAN_POINT('',(-0.49396390682824,-0.000458628609927681,-0.203567954534311));
#65181=CARTESIAN_POINT('Ctrl Pts',(-0.253382212491106,0.424300712223197,
-0.12));
#65182=CARTESIAN_POINT('Ctrl Pts',(-0.183080092417522,0.466283452798211,
-0.122637028314406));
#65183=CARTESIAN_POINT('Ctrl Pts',(-0.0218069960358891,0.513732009672345,
-0.127911084943216));
#65184=CARTESIAN_POINT('Ctrl Pts',(0.310758681059315,0.447140495242652,
-0.138459198200843));
#65185=CARTESIAN_POINT('Ctrl Pts',(0.579077760680187,0.0710394712093248,
-0.151644339772866));
#65186=CARTESIAN_POINT('Ctrl Pts',(0.374813391339547,-0.447521999574274,
-0.167466509659305));
#65187=CARTESIAN_POINT('Ctrl Pts',(-0.170557872637833,-0.557786202019076,
-0.183288679545736));
#65188=CARTESIAN_POINT('Ctrl Pts',(-0.467287313083341,-0.25627684446579,
-0.195322494504073));
#65189=CARTESIAN_POINT('Ctrl Pts',(-0.494353707556968,-0.0466364371496805,
-0.202082252833598));
#65190=CARTESIAN_POINT('Ctrl Pts',(-0.49396390682824,-0.000458628609927681,
-0.203567954534311));
#65191=CARTESIAN_POINT('',(-0.493537605131362,0.000254761609798343,-0.303567954534311));
#65192=CARTESIAN_POINT('Ctrl Pts',(-0.49396390682824,-0.000458628609927681,
-0.203567954534311));
#65193=CARTESIAN_POINT('Ctrl Pts',(-0.492969963352949,0.117289051470408,
-0.207356309462409));
#65194=CARTESIAN_POINT('Ctrl Pts',(-0.392003835461347,0.400544594774385,
-0.21641872101932));
#65195=CARTESIAN_POINT('Ctrl Pts',(0.0799333386512568,0.577918330084977,
-0.230755189205039));
#65196=CARTESIAN_POINT('Ctrl Pts',(0.5280611079658,0.248119757234704,-0.246577359091475));
#65197=CARTESIAN_POINT('Ctrl Pts',(0.495900283769359,-0.307401514562771,
-0.26239952897791));
#65198=CARTESIAN_POINT('Ctrl Pts',(0.0126918090925729,-0.583302937513682,
-0.278221698864343));
#65199=CARTESIAN_POINT('Ctrl Pts',(-0.416412681034692,-0.362461323671283,
-0.291944507383144));
#65200=CARTESIAN_POINT('Ctrl Pts',(-0.493071761030911,-0.0986317868095975,
-0.300393259273133));
#65201=CARTESIAN_POINT('Ctrl Pts',(-0.493537605131362,0.000254761609798343,
-0.303567954534311));
#65202=CARTESIAN_POINT('',(-0.494874876107118,0.000221385223355512,-0.403567954534311));
#65203=CARTESIAN_POINT('Ctrl Pts',(-0.493537605131362,0.000254761609798343,
-0.303567954534311));
#65204=CARTESIAN_POINT('Ctrl Pts',(-0.493845658354544,0.0656464236281961,
-0.305667315901945));
#65205=CARTESIAN_POINT('Ctrl Pts',(-0.451402068223567,0.294932643527596,
-0.313040733898388));
#65206=CARTESIAN_POINT('Ctrl Pts',(-0.104993157557767,0.57391933243674,
-0.325688208523647));
#65207=CARTESIAN_POINT('Ctrl Pts',(0.423865099612549,0.400931541670995,
-0.341510378410082));
#65208=CARTESIAN_POINT('Ctrl Pts',(0.567198827523238,-0.136722713111685,
-0.357332548296515));
#65209=CARTESIAN_POINT('Ctrl Pts',(0.194639240804606,-0.550020940519229,
-0.373154718182949));
#65210=CARTESIAN_POINT('Ctrl Pts',(-0.340699208879849,-0.465305939894536,
-0.388566520262216));
#65211=CARTESIAN_POINT('Ctrl Pts',(-0.494030155161132,-0.150226124138736,
-0.398704265712668));
#65212=CARTESIAN_POINT('Ctrl Pts',(-0.494874876107118,0.000221385223355512,
-0.403567954534311));
#65213=CARTESIAN_POINT('',(-0.494154610429637,-0.000443820138194773,-0.503567954534311));
#65214=CARTESIAN_POINT('Ctrl Pts',(-0.494874876107118,0.000221385223355512,
-0.403567954534311));
#65215=CARTESIAN_POINT('Ctrl Pts',(-0.494946148405776,0.0129152101729008,
-0.40397832234148));
#65216=CARTESIAN_POINT('Ctrl Pts',(-0.488762631718723,0.1886798315986,-0.409662746777461));
#65217=CARTESIAN_POINT('Ctrl Pts',(-0.279363609231548,0.512214322021286,
-0.420621227842251));
#65218=CARTESIAN_POINT('Ctrl Pts',(0.27706667089454,0.513460431776094,-0.436443397728689));
#65219=CARTESIAN_POINT('Ctrl Pts',(0.58149216890127,0.0476908023280638,
-0.45226556761512));
#65220=CARTESIAN_POINT('Ctrl Pts',(0.357023961520341,-0.461455771170997,
-0.468087737501555));
#65221=CARTESIAN_POINT('Ctrl Pts',(-0.192173816477921,-0.550887266295114,
-0.48390990738799));
#65222=CARTESIAN_POINT('Ctrl Pts',(-0.472035147994241,-0.243205736814157,
-0.495736646398908));
#65223=CARTESIAN_POINT('Ctrl Pts',(-0.494512371951871,-0.0401451165327019,
-0.502289328781015));
#65224=CARTESIAN_POINT('Ctrl Pts',(-0.494154610429637,-0.000443820138194773,
-0.503567954534311));
#65225=CARTESIAN_POINT('',(-0.493923623855364,0.000162705886329681,-0.603567957626487));
#65226=CARTESIAN_POINT('Ctrl Pts',(-0.494154610429637,-0.000443820138194773,
-0.503567954534311));
#65227=CARTESIAN_POINT('Ctrl Pts',(-0.493036682507162,0.123614204662111,
-0.507563385409827));
#65228=CARTESIAN_POINT('Ctrl Pts',(-0.382981343090829,0.413199679253085,
-0.516832872914155));
#65229=CARTESIAN_POINT('Ctrl Pts',(0.10242155967994,0.574384395972835,-0.531376417047293));
#65230=CARTESIAN_POINT('Ctrl Pts',(0.537342980930237,0.227310898597556,
-0.547198586933727));
#65231=CARTESIAN_POINT('Ctrl Pts',(0.483525636177959,-0.326511749309766,
-0.563020756820162));
#65232=CARTESIAN_POINT('Ctrl Pts',(-0.0100788586177245,-0.583357998977174,
-0.578842926706596));
#65233=CARTESIAN_POINT('Ctrl Pts',(-0.423901001261801,-0.349516357851695,
-0.592358659277979));
#65234=CARTESIAN_POINT('Ctrl Pts',(-0.493178983690631,-0.0923124040730076,
-0.60060033522055));
#65235=CARTESIAN_POINT('Ctrl Pts',(-0.493454077256828,0.000162454800537643,
-0.60356795453431));
#65236=CARTESIAN_POINT('Ctrl Pts',(-0.494199973167426,0.00016285366162209,
-0.603567959446373));
#65237=CARTESIAN_POINT('Ctrl Pts',(-0.494191229533384,0.0266965137958892,
-0.604418169378795));
#65238=CARTESIAN_POINT('Ctrl Pts',(-0.492041366961323,0.0531673311879112,
-0.605268379311217));
#65239=CARTESIAN_POINT('Ctrl Pts',(-0.487805636429523,0.0792420410362358,
-0.606118589243638));
#65240=CARTESIAN_POINT('Ctrl Pts',(-0.483545285296569,0.105468312705251,
-0.606973741105082));
#65241=CARTESIAN_POINT('Ctrl Pts',(-0.477174931701992,0.131293374138508,
-0.607828892966525));
#65242=CARTESIAN_POINT('Ctrl Pts',(-0.468800804875319,0.156395157687997,
-0.608684044827968));
#65243=CARTESIAN_POINT('Ctrl Pts',(-0.462914752160757,0.174038838546902,
-0.6092851187118));
#65244=CARTESIAN_POINT('Ctrl Pts',(-0.456039796877744,0.191325538833742,
-0.609886192595632));
#65245=CARTESIAN_POINT('Ctrl Pts',(-0.448226612564715,0.20815029134921,
-0.610487266479464));
#65246=CARTESIAN_POINT('Ctrl Pts',(-0.437966149383268,0.230244964507506,
-0.611276611285282));
#65247=CARTESIAN_POINT('Ctrl Pts',(-0.426039665523985,0.251640350874873,
-0.6120659560911));
#65248=CARTESIAN_POINT('Ctrl Pts',(-0.412565452518453,0.272072393653315,
-0.612855300896918));
#65249=CARTESIAN_POINT('Ctrl Pts',(-0.399114683965311,0.292468885705791,
-0.613643272282506));
#65250=CARTESIAN_POINT('Ctrl Pts',(-0.384121865758108,0.311904759778303,
-0.614431243668095));
#65251=CARTESIAN_POINT('Ctrl Pts',(-0.367751076835709,0.330140554137441,
-0.615219215053683));
#65252=CARTESIAN_POINT('Ctrl Pts',(-0.351397634154326,0.348357026123933,
-0.616006351516677));
#65253=CARTESIAN_POINT('Ctrl Pts',(-0.333669560200077,0.36537541101292,
-0.61679348797967));
#65254=CARTESIAN_POINT('Ctrl Pts',(-0.314771364395952,0.380989013170079,
-0.617580624442664));
#65255=CARTESIAN_POINT('Ctrl Pts',(-0.295864722284549,0.396609593627331,
-0.618368112706248));
#65256=CARTESIAN_POINT('Ctrl Pts',(-0.275787434261984,0.41082367793531,
-0.619155600969831));
#65257=CARTESIAN_POINT('Ctrl Pts',(-0.254778215899747,0.423463930816949,
-0.619943089233415));
#65258=CARTESIAN_POINT('Ctrl Pts',(-0.233765382240666,0.436106358851683,
-0.620730713009124));
#65259=CARTESIAN_POINT('Ctrl Pts',(-0.211820907179082,0.447174080969499,
-0.621518336784833));
#65260=CARTESIAN_POINT('Ctrl Pts',(-0.18920904419388,0.456545263468189,
-0.622305960560542));
#65261=CARTESIAN_POINT('Ctrl Pts',(-0.166547864377789,0.465936884664161,
-0.623095302156166));
#65262=CARTESIAN_POINT('Ctrl Pts',(-0.143217046425942,0.473624346369207,
-0.623884643751791));
#65263=CARTESIAN_POINT('Ctrl Pts',(-0.119498511422257,0.479534926535977,
-0.624673985347415));
#65264=CARTESIAN_POINT('Ctrl Pts',(-0.103117558636715,0.483617005578042,
-0.62521913568691));
#65265=CARTESIAN_POINT('Ctrl Pts',(-0.0865520094296256,0.486852600934384,
-0.625764286026405));
#65266=CARTESIAN_POINT('Ctrl Pts',(-0.0698965878358467,0.48923216064452,
-0.6263094363659));
#65267=CARTESIAN_POINT('Ctrl Pts',(-0.0457862380653544,0.492676805776325,
-0.627098594736267));
#65268=CARTESIAN_POINT('Ctrl Pts',(-0.0213536736036407,0.494344433489065,
-0.627887753106634));
#65269=CARTESIAN_POINT('Ctrl Pts',(0.00311537835969982,0.494190180414055,
-0.628676911477001));
#65270=CARTESIAN_POINT('Ctrl Pts',(0.0275418356991093,0.494036195855852,
-0.629464696116009));
#65271=CARTESIAN_POINT('Ctrl Pts',(0.0520039677474236,0.492066577542858,
-0.630252480755017));
#65272=CARTESIAN_POINT('Ctrl Pts',(0.0762116868837025,0.488288253782886,
-0.631040265394026));
#65273=CARTESIAN_POINT('Ctrl Pts',(0.100393757474185,0.484513933229886,
-0.631827215359999));
#65274=CARTESIAN_POINT('Ctrl Pts',(0.124321263762377,0.478934791172687,
-0.632614165325973));
#65275=CARTESIAN_POINT('Ctrl Pts',(0.147709532962699,0.471609514187258,
-0.633401115291947));
#65276=CARTESIAN_POINT('Ctrl Pts',(0.171108332587079,0.464280939041014,
-0.634188419577292));
#65277=CARTESIAN_POINT('Ctrl Pts',(0.193966740932735,0.455204844567866,
-0.634975723862637));
#65278=CARTESIAN_POINT('Ctrl Pts',(0.216014424973876,0.444490054110557,
-0.635763028147983));
#65279=CARTESIAN_POINT('Ctrl Pts',(0.238065935515635,0.43377340404059,-0.636550469074453));
#65280=CARTESIAN_POINT('Ctrl Pts',(0.259305828612904,0.421417819004453,
-0.637337910000922));
#65281=CARTESIAN_POINT('Ctrl Pts',(0.279487991968314,0.407578338906179,
-0.638125350927392));
#65282=CARTESIAN_POINT('Ctrl Pts',(0.299714305925911,0.393708583491549,
-0.638914514463598));
#65283=CARTESIAN_POINT('Ctrl Pts',(0.318877717704755,0.37834887532309,-0.639703677999804));
#65284=CARTESIAN_POINT('Ctrl Pts',(0.336763654525841,0.361695840438344,
-0.640492841536009));
#65285=CARTESIAN_POINT('Ctrl Pts',(0.349144207197986,0.35016869609002,-0.641039096441451));
#65286=CARTESIAN_POINT('Ctrl Pts',(0.360913380964598,0.338022736759383,
-0.641585351346892));
#65287=CARTESIAN_POINT('Ctrl Pts',(0.372011165225625,0.325332649679482,
-0.642131606252334));
#65288=CARTESIAN_POINT('Ctrl Pts',(0.388048694568756,0.306994066127674,
-0.642921005187183));
#65289=CARTESIAN_POINT('Ctrl Pts',(0.402771380822854,0.287415961485453,
-0.643710404122033));
#65290=CARTESIAN_POINT('Ctrl Pts',(0.415985784972064,0.266813542949334,
-0.644499803056882));
#65291=CARTESIAN_POINT('Ctrl Pts',(0.429177169125266,0.246247014612053,
-0.64528782682868));
#65292=CARTESIAN_POINT('Ctrl Pts',(0.440865072248985,0.224660263493484,
-0.646075850600479));
#65293=CARTESIAN_POINT('Ctrl Pts',(0.450897100945209,0.202300381510282,
-0.646863874372277));
#65294=CARTESIAN_POINT('Ctrl Pts',(0.460918476799838,0.179964243107574,
-0.647651061354961));
#65295=CARTESIAN_POINT('Ctrl Pts',(0.469287161597707,0.15685722216568,-0.648438248337644));
#65296=CARTESIAN_POINT('Ctrl Pts',(0.475897104792094,0.133250086868651,
-0.649225435320328));
#65297=CARTESIAN_POINT('Ctrl Pts',(0.482509973753802,0.109632502316165,
-0.650012970736558));
#65298=CARTESIAN_POINT('Ctrl Pts',(0.487362337295631,0.0855150232019731,
-0.650800506152787));
#65299=CARTESIAN_POINT('Ctrl Pts',(0.490397992575441,0.0611837305006642,
-0.651588041569017));
#65300=CARTESIAN_POINT('Ctrl Pts',(0.493434163220453,0.0368483070597128,
-0.652375710685655));
#65301=CARTESIAN_POINT('Ctrl Pts',(0.494652951573273,0.0122996895892027,
-0.653163379802293));
#65302=CARTESIAN_POINT('Ctrl Pts',(0.494050102097953,-0.0121711386896278,
-0.653951048918932));
#65303=CARTESIAN_POINT('Ctrl Pts',(0.493445940628029,-0.0366952233715363,
-0.654740432257233));
#65304=CARTESIAN_POINT('Ctrl Pts',(0.491012279604423,-0.0611404871652856,
-0.655529815595535));
#65305=CARTESIAN_POINT('Ctrl Pts',(0.486796920891336,-0.0852197031836814,
-0.656319198933837));
#65306=CARTESIAN_POINT('Ctrl Pts',(0.48388733779075,-0.101839992172365,
-0.656864058002148));
#65307=CARTESIAN_POINT('Ctrl Pts',(0.480130017358319,-0.118286007874321,
-0.657408917070458));
#65308=CARTESIAN_POINT('Ctrl Pts',(0.475554570486741,-0.13446743281989,
-0.657953776138768));
#65309=CARTESIAN_POINT('Ctrl Pts',(0.468924039663125,-0.157916822547936,
-0.658743361276211));
#65310=CARTESIAN_POINT('Ctrl Pts',(0.460536659523053,-0.180939245255025,
-0.659532946413655));
#65311=CARTESIAN_POINT('Ctrl Pts',(0.450467533895641,-0.203255112865531,
-0.660322531551098));
#65312=CARTESIAN_POINT('Ctrl Pts',(0.440415891764968,-0.225532232384789,
-0.661110745694704));
#65313=CARTESIAN_POINT('Ctrl Pts',(0.428688535079481,-0.247104585693906,
-0.66189895983831));
#65314=CARTESIAN_POINT('Ctrl Pts',(0.415409667071266,-0.267709634686053,
-0.662687173981916));
#65315=CARTESIAN_POINT('Ctrl Pts',(0.402144836964618,-0.288292900823717,
-0.66347455485626));
#65316=CARTESIAN_POINT('Ctrl Pts',(0.387332102670531,-0.307910298342129,
-0.664261935730603));
#65317=CARTESIAN_POINT('Ctrl Pts',(0.371140771576259,-0.326325248293446,
-0.665049316604946));
#65318=CARTESIAN_POINT('Ctrl Pts',(0.354942213600477,-0.34474841762219,
-0.665837048920949));
#65319=CARTESIAN_POINT('Ctrl Pts',(0.337364270730379,-0.361967531821357,
-0.666624781236952));
#65320=CARTESIAN_POINT('Ctrl Pts',(0.318616254647902,-0.377779462483263,
-0.667412513552956));
#65321=CARTESIAN_POINT('Ctrl Pts',(0.299865009486434,-0.393594116525226,
-0.668200381544641));
#65322=CARTESIAN_POINT('Ctrl Pts',(0.279943836914778,-0.408000677387485,
-0.668988249536327));
#65323=CARTESIAN_POINT('Ctrl Pts',(0.259094471956554,-0.420836897861338,
-0.669776117528012));
#65324=CARTESIAN_POINT('Ctrl Pts',(0.238199748108907,-0.433701044207574,
-0.670565699567929));
#65325=CARTESIAN_POINT('Ctrl Pts',(0.216373410584568,-0.444987696202054,
-0.671355281607845));
#65326=CARTESIAN_POINT('Ctrl Pts',(0.193882421600628,-0.45458029719102,
-0.672144863647761));
#65327=CARTESIAN_POINT('Ctrl Pts',(0.178395470307243,-0.461185615632067,
-0.672688557773575));
#65328=CARTESIAN_POINT('Ctrl Pts',(0.162593874688042,-0.466988692461513,
-0.673232251899389));
#65329=CARTESIAN_POINT('Ctrl Pts',(0.146568870670712,-0.471965259473949,
-0.673775946025203));
#65330=CARTESIAN_POINT('Ctrl Pts',(0.123334115400948,-0.479180815644323,
-0.674564251596997));
#65331=CARTESIAN_POINT('Ctrl Pts',(0.099499908992319,-0.484696776467554,
-0.675352557168792));
#65332=CARTESIAN_POINT('Ctrl Pts',(0.0753406616753785,-0.488423407197399,
-0.676140862740586));
#65333=CARTESIAN_POINT('Ctrl Pts',(0.0512235350854168,-0.49214354068859,
-0.676927793931659));
#65334=CARTESIAN_POINT('Ctrl Pts',(0.0267831641950888,-0.494080378759341,
-0.677714725122732));
#65335=CARTESIAN_POINT('Ctrl Pts',(0.00230653230264751,-0.494194617442093,
-0.678501656313805));
#65336=CARTESIAN_POINT('Ctrl Pts',(-0.0221441954689344,-0.494308735223708,
-0.679287754679481));
#65337=CARTESIAN_POINT('Ctrl Pts',(-0.0466304160046617,-0.49260405195665,
-0.680073853045156));
#65338=CARTESIAN_POINT('Ctrl Pts',(-0.0708622501506096,-0.4890932237351,
-0.680859951410832));
#65339=CARTESIAN_POINT('Ctrl Pts',(-0.0951053905960956,-0.485580757400839,
-0.681646416561107));
#65340=CARTESIAN_POINT('Ctrl Pts',(-0.119093215612431,-0.480260540258949,
-0.682432881711382));
#65341=CARTESIAN_POINT('Ctrl Pts',(-0.142542033323854,-0.4731970083759,
-0.683219346861658));
#65342=CARTESIAN_POINT('Ctrl Pts',(-0.165995093287149,-0.466132198591264,
-0.684005954295578));
#65343=CARTESIAN_POINT('Ctrl Pts',(-0.188908293129803,-0.457323672770647,
-0.684792561729498));
#65344=CARTESIAN_POINT('Ctrl Pts',(-0.211014537655382,-0.446885337528639,
-0.685579169163419));
#65345=CARTESIAN_POINT('Ctrl Pts',(-0.233169828021835,-0.436423843358452,
-0.686367521797569));
#65346=CARTESIAN_POINT('Ctrl Pts',(-0.254513974367191,-0.424325651739701,
-0.68715587443172));
#65347=CARTESIAN_POINT('Ctrl Pts',(-0.27480444503967,-0.410750723659057,
-0.68794422706587));
#65348=CARTESIAN_POINT('Ctrl Pts',(-0.288993604250444,-0.401257754327777,
-0.688495523347792));
#65349=CARTESIAN_POINT('Ctrl Pts',(-0.302668046169075,-0.391043594242111,
-0.689046819629715));
#65350=CARTESIAN_POINT('Ctrl Pts',(-0.315754697256002,-0.380174448327042,
-0.689598115911637));
#65351=CARTESIAN_POINT('Ctrl Pts',(-0.334269196694398,-0.364797191410533,
-0.690378069058874));
#65352=CARTESIAN_POINT('Ctrl Pts',(-0.351715095282875,-0.348016403869801,
-0.691158022206111));
#65353=CARTESIAN_POINT('Ctrl Pts',(-0.367870045722719,-0.330007983933668,
-0.691937975353348));
#65354=CARTESIAN_POINT('Ctrl Pts',(-0.383996609505757,-0.312031207476621,
-0.692716558006606));
#65355=CARTESIAN_POINT('Ctrl Pts',(-0.398836213732678,-0.292831564643769,
-0.693495140659864));
#65356=CARTESIAN_POINT('Ctrl Pts',(-0.41220165015197,-0.272623255816508,
-0.694273723313121));
#65357=CARTESIAN_POINT('Ctrl Pts',(-0.425561954706966,-0.252422706279352,
-0.695052007017628));
#65358=CARTESIAN_POINT('Ctrl Pts',(-0.437448782125241,-0.2312148239441,
-0.695830290722135));
#65359=CARTESIAN_POINT('Ctrl Pts',(-0.44771653219203,-0.209245183461753,
-0.696608574426642));
#65360=CARTESIAN_POINT('Ctrl Pts',(-0.457980502294138,-0.187283630872522,
-0.697386571614152));
#65361=CARTESIAN_POINT('Ctrl Pts',(-0.466626279375811,-0.164561523677347,
-0.698164568801661));
#65362=CARTESIAN_POINT('Ctrl Pts',(-0.473555426179341,-0.141346730899949,
-0.698942565989171));
#65363=CARTESIAN_POINT('Ctrl Pts',(-0.480497095026677,-0.118089985388637,
-0.699721969138358));
#65364=CARTESIAN_POINT('Ctrl Pts',(-0.485715746205358,-0.0943394653797793,
-0.700501372287546));
#65365=CARTESIAN_POINT('Ctrl Pts',(-0.489163270445009,-0.0703770903600209,
-0.701280775436733));
#65366=CARTESIAN_POINT('Ctrl Pts',(-0.492535554042889,-0.0469376832295417,
-0.702043168468205));
#65367=CARTESIAN_POINT('Ctrl Pts',(-0.494213349678348,-0.0232962356163744,
-0.702805561499676));
#65368=CARTESIAN_POINT('Ctrl Pts',(-0.494199919830197,0.000281495695726313,
-0.703567954531148));
#65369=CARTESIAN_POINT('Origin',(0.,0.,-0.920658989190502));
#65370=CARTESIAN_POINT('',(-0.437199811556163,-0.000405925184154985,-0.170658989186969));
#65371=CARTESIAN_POINT('Ctrl Pts',(-0.00922985932074797,0.43710256198851,
-0.195314102181071));
#65372=CARTESIAN_POINT('Ctrl Pts',(-0.0315222221120698,0.436631836373096,
-0.194501442586441));
#65373=CARTESIAN_POINT('Ctrl Pts',(-0.0538211649838741,0.434450494946843,
-0.193688782991811));
#65374=CARTESIAN_POINT('Ctrl Pts',(-0.0758452307453741,0.430570947665052,
-0.192876123397182));
#65375=CARTESIAN_POINT('Ctrl Pts',(-0.0978465938203715,0.426695399469836,
-0.192064301502376));
#65376=CARTESIAN_POINT('Ctrl Pts',(-0.119572937063035,0.421125217966566,
-0.19125247960757));
#65377=CARTESIAN_POINT('Ctrl Pts',(-0.140749458739654,0.413924425305507,
-0.190440657712765));
#65378=CARTESIAN_POINT('Ctrl Pts',(-0.161936626482776,0.406720012592076,
-0.189628427690977));
#65379=CARTESIAN_POINT('Ctrl Pts',(-0.182572738074923,0.397883565095202,
-0.188816197669189));
#65380=CARTESIAN_POINT('Ctrl Pts',(-0.202398840300782,0.387528772409093,
-0.188003967647401));
#65381=CARTESIAN_POINT('Ctrl Pts',(-0.222230291718209,0.377171185942891,
-0.187191518481481));
#65382=CARTESIAN_POINT('Ctrl Pts',(-0.24125068040462,0.365294798452339,
-0.18637906931556));
#65383=CARTESIAN_POINT('Ctrl Pts',(-0.259226882313261,0.352058608027338,
-0.185566620149639));
#65384=CARTESIAN_POINT('Ctrl Pts',(-0.277241404192072,0.338794201941163,
-0.184752439081286));
#65385=CARTESIAN_POINT('Ctrl Pts',(-0.294206749929414,0.324164669578954,
-0.183938258012934));
#65386=CARTESIAN_POINT('Ctrl Pts',(-0.309923124603311,0.308369091894957,
-0.183124076944581));
#65387=CARTESIAN_POINT('Ctrl Pts',(-0.317001146030817,0.301255400625376,
-0.18275740262132));
#65388=CARTESIAN_POINT('Ctrl Pts',(-0.32382636374821,0.293905688877171,
-0.182390728298059));
#65389=CARTESIAN_POINT('Ctrl Pts',(-0.330383231586033,0.286340287571919,
-0.182024053974797));
#65390=CARTESIAN_POINT('Ctrl Pts',(-0.344802295372176,0.269703380029126,
-0.181217708538743));
#65391=CARTESIAN_POINT('Ctrl Pts',(-0.358007064617044,0.251921858419598,
-0.180411363102688));
#65392=CARTESIAN_POINT('Ctrl Pts',(-0.369812380149333,0.233200865110499,
-0.179605017666633));
#65393=CARTESIAN_POINT('Ctrl Pts',(-0.381596643628483,0.214513256368282,
-0.178800110161392));
#65394=CARTESIAN_POINT('Ctrl Pts',(-0.39198596824022,0.194890077933115,
-0.17799520265615));
#65395=CARTESIAN_POINT('Ctrl Pts',(-0.400836298367205,0.174568330207047,
-0.177190295150909));
#65396=CARTESIAN_POINT('Ctrl Pts',(-0.409677025326455,0.154268632862072,
-0.1763862610212));
#65397=CARTESIAN_POINT('Ctrl Pts',(-0.4169817556723,0.133272525650334,-0.175582226891491));
#65398=CARTESIAN_POINT('Ctrl Pts',(-0.422653074331143,0.111840148240392,
-0.174778192761782));
#65399=CARTESIAN_POINT('Ctrl Pts',(-0.428326882958909,0.0903983610340917,
-0.173973805624225));
#65400=CARTESIAN_POINT('Ctrl Pts',(-0.432365646160191,0.0685206233884101,
-0.173169418486668));
#65401=CARTESIAN_POINT('Ctrl Pts',(-0.434722135461347,0.0464812321257325,
-0.172365031349111));
#65402=CARTESIAN_POINT('Ctrl Pts',(-0.436388111915708,0.030899957517756,
-0.171796350629574));
#65403=CARTESIAN_POINT('Ctrl Pts',(-0.437214336588321,0.0152381961726338,
-0.171227669910038));
#65404=CARTESIAN_POINT('Ctrl Pts',(-0.437199811556254,-0.000405925086964313,
-0.170658989190502));
#65405=CARTESIAN_POINT('',(0.43681045027439,0.0184518435687243,-0.120000432818402));
#65406=CARTESIAN_POINT('Ctrl Pts',(-0.437199811556163,-0.000405925184156353,
-0.170658989186969));
#65407=CARTESIAN_POINT('Ctrl Pts',(-0.437174206827099,-0.0279833782682871,
-0.169656518955322));
#65408=CARTESIAN_POINT('Ctrl Pts',(-0.434535377857394,-0.0554441171566531,
-0.168654048723676));
#65409=CARTESIAN_POINT('Ctrl Pts',(-0.429372126588209,-0.0823615013772751,
-0.16765157849203));
#65410=CARTESIAN_POINT('Ctrl Pts',(-0.426883229251288,-0.0953367765306281,
-0.167168347024141));
#65411=CARTESIAN_POINT('Ctrl Pts',(-0.423808466932811,-0.108186137755551,
-0.166685115556252));
#65412=CARTESIAN_POINT('Ctrl Pts',(-0.420161672749106,-0.120863595646799,
-0.166201884088363));
#65413=CARTESIAN_POINT('Ctrl Pts',(-0.414011914527358,-0.142242181048175,
-0.165386988444969));
#65414=CARTESIAN_POINT('Ctrl Pts',(-0.406208909896096,-0.163210776284862,
-0.164572092801575));
#65415=CARTESIAN_POINT('Ctrl Pts',(-0.396827640688903,-0.183498402132766,
-0.16375719715818));
#65416=CARTESIAN_POINT('Ctrl Pts',(-0.387463194782531,-0.203749646460747,
-0.162943762855916));
#65417=CARTESIAN_POINT('Ctrl Pts',(-0.376526348646218,-0.223321681805135,
-0.162130328553652));
#65418=CARTESIAN_POINT('Ctrl Pts',(-0.364140998075861,-0.241961099188105,
-0.161316894251388));
#65419=CARTESIAN_POINT('Ctrl Pts',(-0.351768955503626,-0.260580488608998,
-0.160504333980271));
#65420=CARTESIAN_POINT('Ctrl Pts',(-0.337951868176142,-0.278268642824925,
-0.159691773709154));
#65421=CARTESIAN_POINT('Ctrl Pts',(-0.322858308296458,-0.294798834400595,
-0.158879213438037));
#65422=CARTESIAN_POINT('Ctrl Pts',(-0.307758065787926,-0.311336344669533,
-0.158066293408272));
#65423=CARTESIAN_POINT('Ctrl Pts',(-0.291380688599474,-0.32671432818191,
-0.157253373378506));
#65424=CARTESIAN_POINT('Ctrl Pts',(-0.273933983018575,-0.340740389369354,
-0.156440453348741));
#65425=CARTESIAN_POINT('Ctrl Pts',(-0.256483336968056,-0.354769618448165,
-0.155627349714875));
#65426=CARTESIAN_POINT('Ctrl Pts',(-0.237963456582662,-0.367445893883955,
-0.154814246081008));
#65427=CARTESIAN_POINT('Ctrl Pts',(-0.218613434383194,-0.378618549872012,
-0.154001142447142));
#65428=CARTESIAN_POINT('Ctrl Pts',(-0.199222816794282,-0.389814645539686,
-0.153186332962072));
#65429=CARTESIAN_POINT('Ctrl Pts',(-0.178999221425296,-0.399500507709868,
-0.152371523477002));
#65430=CARTESIAN_POINT('Ctrl Pts',(-0.158205278778461,-0.407571993354094,
-0.151556713991931));
#65431=CARTESIAN_POINT('Ctrl Pts',(-0.148192931689111,-0.411458438419815,
-0.151164380728597));
#65432=CARTESIAN_POINT('Ctrl Pts',(-0.13804861769082,-0.414971330636069,
-0.150772047465263));
#65433=CARTESIAN_POINT('Ctrl Pts',(-0.127802767782729,-0.418103208008589,
-0.150379714201928));
#65434=CARTESIAN_POINT('Ctrl Pts',(-0.106505478982892,-0.424613209373686,
-0.149564200126477));
#65435=CARTESIAN_POINT('Ctrl Pts',(-0.0846507791638919,-0.429509775307143,
-0.148748686051025));
#65436=CARTESIAN_POINT('Ctrl Pts',(-0.0625073938790264,-0.432708522807735,
-0.147933171975573));
#65437=CARTESIAN_POINT('Ctrl Pts',(-0.0404028108791555,-0.435901665080827,
-0.147119086941308));
#65438=CARTESIAN_POINT('Ctrl Pts',(-0.0180112363006184,-0.437402741450067,
-0.146305001907042));
#65439=CARTESIAN_POINT('Ctrl Pts',(0.00438680710504075,-0.437177991124237,
-0.145490916872777));
#65440=CARTESIAN_POINT('Ctrl Pts',(0.0267616142569755,-0.436953473959647,
-0.144677676389353));
#65441=CARTESIAN_POINT('Ctrl Pts',(0.0491421680956022,-0.435006665496692,
-0.143864435905929));
#65442=CARTESIAN_POINT('Ctrl Pts',(0.0712460812121622,-0.431355811264796,
-0.143051195422505));
#65443=CARTESIAN_POINT('Ctrl Pts',(0.093360723961109,-0.427703184843351,
-0.142237560177693));
#65444=CARTESIAN_POINT('Ctrl Pts',(0.115197752260316,-0.422344958720878,
-0.14142392493288));
#65445=CARTESIAN_POINT('Ctrl Pts',(0.136482264438377,-0.415350973868815,
-0.140610289688068));
#65446=CARTESIAN_POINT('Ctrl Pts',(0.157772123242929,-0.408355232141876,
-0.139796450059725));
#65447=CARTESIAN_POINT('Ctrl Pts',(0.178508523103308,-0.399723165427198,
-0.138982610431382));
#65448=CARTESIAN_POINT('Ctrl Pts',(0.198434570732757,-0.389573563191994,
-0.138168770803039));
#65449=CARTESIAN_POINT('Ctrl Pts',(0.218402865165291,-0.379402441975454,
-0.137353205688379));
#65450=CARTESIAN_POINT('Ctrl Pts',(0.23755676455108,-0.367707726858595,
-0.13653764057372));
#65451=CARTESIAN_POINT('Ctrl Pts',(0.255665599555166,-0.354653268988314,
-0.13572207545906));
#65452=CARTESIAN_POINT('Ctrl Pts',(0.264284695671018,-0.348439858401775,
-0.135333898411205));
#65453=CARTESIAN_POINT('Ctrl Pts',(0.272667507689819,-0.341919023909054,
-0.13494572136335));
#65454=CARTESIAN_POINT('Ctrl Pts',(0.280791942218824,-0.335111511567389,
-0.134557544315494));
#65455=CARTESIAN_POINT('Ctrl Pts',(0.297492947322032,-0.321117639384359,
-0.133759587628905));
#65456=CARTESIAN_POINT('Ctrl Pts',(0.313202957866233,-0.305823455159743,
-0.132961630942315));
#65457=CARTESIAN_POINT('Ctrl Pts',(0.327708795017198,-0.289397279994779,
-0.132163674255725));
#65458=CARTESIAN_POINT('Ctrl Pts',(0.342188440452228,-0.273000763904939,
-0.131367158358429));
#65459=CARTESIAN_POINT('Ctrl Pts',(0.35546768938981,-0.255476819080919,
-0.130570642461133));
#65460=CARTESIAN_POINT('Ctrl Pts',(0.367368586639539,-0.237031984235182,
-0.129774126563837));
#65461=CARTESIAN_POINT('Ctrl Pts',(0.379537806510062,-0.218171284406993,
-0.128959652085051));
#65462=CARTESIAN_POINT('Ctrl Pts',(0.390265160915261,-0.198348215478529,
-0.128145177606265));
#65463=CARTESIAN_POINT('Ctrl Pts',(0.399405653984382,-0.177817219541044,
-0.127330703127478));
#65464=CARTESIAN_POINT('Ctrl Pts',(0.408340170441622,-0.15774887971519,
-0.126534582439055));
#65465=CARTESIAN_POINT('Ctrl Pts',(0.415758405797366,-0.137004945668643,
-0.125738461750631));
#65466=CARTESIAN_POINT('Ctrl Pts',(0.421573066228182,-0.115844679769807,
-0.124942341062208));
#65467=CARTESIAN_POINT('Ctrl Pts',(0.427588803694421,-0.0939526697585951,
-0.12411868968824));
#65468=CARTESIAN_POINT('Ctrl Pts',(0.43188766654941,-0.0716157931141208,
-0.123295038314273));
#65469=CARTESIAN_POINT('Ctrl Pts',(0.43443041023611,-0.0491330709612701,
-0.122471386940305));
#65470=CARTESIAN_POINT('Ctrl Pts',(0.43697315392281,-0.0266503488084183,
-0.121647735566337));
#65471=CARTESIAN_POINT('Ctrl Pts',(0.437759823048745,-0.00402265593044939,
-0.12082408419237));
#65472=CARTESIAN_POINT('Ctrl Pts',(0.43681045027439,0.0184518435687243,
-0.120000432818402));
#65473=CARTESIAN_POINT('',(0.159436307123189,-0.407092009220176,-0.12));
#65474=CARTESIAN_POINT('Origin',(0.,0.,-0.12));
#65475=CARTESIAN_POINT('',(-0.437199999925775,8.05617700352763E-6,-0.150941010806857));
#65476=CARTESIAN_POINT('Ctrl Pts',(-0.437199999925775,8.05617700357433E-6,
-0.150941010806857));
#65477=CARTESIAN_POINT('Ctrl Pts',(-0.437200411510969,-0.0223282264816288,
-0.150121936742549));
#65478=CARTESIAN_POINT('Ctrl Pts',(-0.435484786799362,-0.0447284246752743,
-0.149302862678242));
#65479=CARTESIAN_POINT('Ctrl Pts',(-0.43204974625499,-0.0669093174453197,
-0.148483788613934));
#65480=CARTESIAN_POINT('Ctrl Pts',(-0.428621461812277,-0.08904658442274,
-0.147666325519736));
#65481=CARTESIAN_POINT('Ctrl Pts',(-0.423480525826266,-0.110964704565275,
-0.146848862425539));
#65482=CARTESIAN_POINT('Ctrl Pts',(-0.41667541902183,-0.132383666601974,
-0.146031399331341));
#65483=CARTESIAN_POINT('Ctrl Pts',(-0.409593050690594,-0.154675304746105,
-0.145180630210932));
#65484=CARTESIAN_POINT('Ctrl Pts',(-0.400707930092937,-0.176425394702839,
-0.144329861090523));
#65485=CARTESIAN_POINT('Ctrl Pts',(-0.390133072634072,-0.197332272163217,
-0.143479091970115));
#65486=CARTESIAN_POINT('Ctrl Pts',(-0.379985497716015,-0.217394396514025,
-0.142662698612483));
#65487=CARTESIAN_POINT('Ctrl Pts',(-0.368282628512785,-0.236679550736123,
-0.141846305254851));
#65488=CARTESIAN_POINT('Ctrl Pts',(-0.355172417599625,-0.254943903195267,
-0.14102991189722));
#65489=CARTESIAN_POINT('Ctrl Pts',(-0.34206142917299,-0.273209338839131,
-0.140213470122607));
#65490=CARTESIAN_POINT('Ctrl Pts',(-0.327543361401381,-0.290453292232999,
-0.139397028347994));
#65491=CARTESIAN_POINT('Ctrl Pts',(-0.3118077799158,-0.306463290434564,
-0.138580586573381));
#65492=CARTESIAN_POINT('Ctrl Pts',(-0.296049869827803,-0.322496006632592,
-0.137762986277629));
#65493=CARTESIAN_POINT('Ctrl Pts',(-0.279071522280868,-0.337290801418832,
-0.136945385981878));
#65494=CARTESIAN_POINT('Ctrl Pts',(-0.261097572399393,-0.350673491566077,
-0.136127785686126));
#65495=CARTESIAN_POINT('Ctrl Pts',(-0.258858041626556,-0.35234095734882,
-0.136025913752896));
#65496=CARTESIAN_POINT('Ctrl Pts',(-0.25660309183787,-0.353986555224397,
-0.135924041819665));
#65497=CARTESIAN_POINT('Ctrl Pts',(-0.254333188587303,-0.355609995898619,
-0.135822169886434));
#65498=CARTESIAN_POINT('Ctrl Pts',(-0.236102803290399,-0.368648414602289,
-0.135004000833075));
#65499=CARTESIAN_POINT('Ctrl Pts',(-0.216831887317712,-0.380306736362932,
-0.134185831779715));
#65500=CARTESIAN_POINT('Ctrl Pts',(-0.196755198149015,-0.390424425467134,
-0.133367662726355));
#65501=CARTESIAN_POINT('Ctrl Pts',(-0.176702518611316,-0.400530014868049,
-0.132550472118042));
#65502=CARTESIAN_POINT('Ctrl Pts',(-0.15584659277195,-0.409098288862712,
-0.131733281509728));
#65503=CARTESIAN_POINT('Ctrl Pts',(-0.134447898286254,-0.416013945254734,
-0.130916090901415));
#65504=CARTESIAN_POINT('Ctrl Pts',(-0.113054594805081,-0.422927859375287,
-0.130099106169131));
#65505=CARTESIAN_POINT('Ctrl Pts',(-0.0911194600821032,-0.428189754850942,
-0.129282121436848));
#65506=CARTESIAN_POINT('Ctrl Pts',(-0.0689198346927786,-0.431733594229034,
-0.128465136704564));
#65507=CARTESIAN_POINT('Ctrl Pts',(-0.0639014865065837,-0.432534698734327,
-0.128280452784115));
#65508=CARTESIAN_POINT('Ctrl Pts',(-0.058869668093171,-0.433248214564207,
-0.128095768863666));
#65509=CARTESIAN_POINT('Ctrl Pts',(-0.0538276487004057,-0.433873742274623,
-0.127911084943217));
#65510=CARTESIAN_POINT('Ctrl Pts',(-0.0281379123489383,-0.437060886295561,
-0.126970096649617));
#65511=CARTESIAN_POINT('Ctrl Pts',(-0.00221150245003065,-0.437956315129622,
-0.126029108356018));
#65512=CARTESIAN_POINT('Ctrl Pts',(0.0235731099185724,-0.436564025646602,
-0.125088120062418));
#65513=CARTESIAN_POINT('Ctrl Pts',(0.0494083253767184,-0.435169003752934,
-0.124145285050543));
#65514=CARTESIAN_POINT('Ctrl Pts',(0.0751009302224881,-0.43147733488461,
-0.123202450038669));
#65515=CARTESIAN_POINT('Ctrl Pts',(0.100276446654969,-0.425544914487593,
-0.122259615026794));
#65516=CARTESIAN_POINT('Ctrl Pts',(0.120388475631987,-0.420805666685124,
-0.121506410017863));
#65517=CARTESIAN_POINT('Ctrl Pts',(0.140170569315508,-0.414637374937239,
-0.120753205008931));
#65518=CARTESIAN_POINT('Ctrl Pts',(0.159436307123189,-0.407092009220176,
-0.12));
#65519=CARTESIAN_POINT('Ctrl Pts',(-0.00922985932074711,0.43710256198851,
-0.175603427251549));
#65520=CARTESIAN_POINT('Ctrl Pts',(-0.0316398144068825,0.436629353293763,
-0.174789798874397));
#65521=CARTESIAN_POINT('Ctrl Pts',(-0.05401454645459,0.434428359633278,
-0.173976170497244));
#65522=CARTESIAN_POINT('Ctrl Pts',(-0.0760722143289932,0.430530902731829,
-0.173162542120091));
#65523=CARTESIAN_POINT('Ctrl Pts',(-0.098137492626593,0.426632101114493,
-0.172348633021681));
#65524=CARTESIAN_POINT('Ctrl Pts',(-0.119884794677085,0.421035830047629,
-0.17153472392327));
#65525=CARTESIAN_POINT('Ctrl Pts',(-0.141043448082782,0.413824341663126,
-0.170720814824859));
#65526=CARTESIAN_POINT('Ctrl Pts',(-0.162246071690038,0.406597866946945,
-0.169905214326414));
#65527=CARTESIAN_POINT('Ctrl Pts',(-0.182856949803843,0.397749755060883,
-0.169089613827968));
#65528=CARTESIAN_POINT('Ctrl Pts',(-0.202625341126216,0.387410391101587,
-0.168274013329523));
#65529=CARTESIAN_POINT('Ctrl Pts',(-0.209149388368132,0.383998150933847,
-0.16800484543945));
#65530=CARTESIAN_POINT('Ctrl Pts',(-0.215581891325189,0.380423853186842,
-0.167735677549376));
#65531=CARTESIAN_POINT('Ctrl Pts',(-0.221914529893185,0.376693219241184,
-0.167466509659303));
#65532=CARTESIAN_POINT('Ctrl Pts',(-0.240883208540412,0.365518541307841,
-0.166660248705969));
#65533=CARTESIAN_POINT('Ctrl Pts',(-0.259065747553711,0.352871957896418,
-0.165853987752634));
#65534=CARTESIAN_POINT('Ctrl Pts',(-0.276221285039249,0.338888833824996,
-0.1650477267993));
#65535=CARTESIAN_POINT('Ctrl Pts',(-0.293345921637636,0.3249308964281,-0.164242918098846));
#65536=CARTESIAN_POINT('Ctrl Pts',(-0.309446629671869,0.309641603187625,
-0.163438109398393));
#65537=CARTESIAN_POINT('Ctrl Pts',(-0.32431133029229,0.293199592503205,
-0.162633300697939));
#65538=CARTESIAN_POINT('Ctrl Pts',(-0.339160503636931,0.276774756711222,
-0.161829332679512));
#65539=CARTESIAN_POINT('Ctrl Pts',(-0.35277572259787,0.259200111547914,
-0.161025364661085));
#65540=CARTESIAN_POINT('Ctrl Pts',(-0.364981679555856,0.240691116555195,
-0.160221396642658));
#65541=CARTESIAN_POINT('Ctrl Pts',(-0.377195275526492,0.22217053783763,
-0.159416925466479));
#65542=CARTESIAN_POINT('Ctrl Pts',(-0.387997430440119,0.202715040834984,
-0.1586124542903));
#65543=CARTESIAN_POINT('Ctrl Pts',(-0.397255788478525,0.182569653886688,
-0.157807983114121));
#65544=CARTESIAN_POINT('Ctrl Pts',(-0.406517033128674,0.162417985920715,
-0.157003261116368));
#65545=CARTESIAN_POINT('Ctrl Pts',(-0.414233252420819,0.141576678642802,
-0.156198539118614));
#65546=CARTESIAN_POINT('Ctrl Pts',(-0.420320381114166,0.120310503365427,
-0.15539381712086));
#65547=CARTESIAN_POINT('Ctrl Pts',(-0.426422168501408,0.0989931160356346,
-0.154587157235141));
#65548=CARTESIAN_POINT('Ctrl Pts',(-0.430886886337158,0.0772495345773366,
-0.153780497349423));
#65549=CARTESIAN_POINT('Ctrl Pts',(-0.433681462773864,0.0553554771122185,
-0.152973837463704));
#65550=CARTESIAN_POINT('Ctrl Pts',(-0.435216757877885,0.0433272359834948,
-0.152530671566759));
#65551=CARTESIAN_POINT('Ctrl Pts',(-0.43624888740812,0.0312536725423513,
-0.152087505669814));
#65552=CARTESIAN_POINT('Ctrl Pts',(-0.436779063571225,0.0191804490521891,
-0.151644339772869));
#65553=CARTESIAN_POINT('Ctrl Pts',(-0.437059536605343,0.0127934896611146,
-0.151409896785079));
#65554=CARTESIAN_POINT('Ctrl Pts',(-0.437199882116983,0.00640135457303683,
-0.151175453797288));
#65555=CARTESIAN_POINT('Ctrl Pts',(-0.437199999925774,8.05624901829692E-6,
-0.150941010809498));
#65556=CARTESIAN_POINT('Origin',(4.51336705371395E-17,0.,-0.12));
#65557=CARTESIAN_POINT('',(0.436962529762211,0.0516115063121503,-0.12));
#65558=CARTESIAN_POINT('Ctrl Pts',(0.43738504590192,0.0184879624732976,
-0.12));
#65559=CARTESIAN_POINT('Ctrl Pts',(0.437692020904658,0.0295490537246066,
-0.12));
#65560=CARTESIAN_POINT('Ctrl Pts',(0.437554515524168,0.0405981455361159,
-0.12));
#65561=CARTESIAN_POINT('Ctrl Pts',(0.436962529762211,0.0516115063121503,
-0.12));
#65562=CARTESIAN_POINT('',(0.118083290997715,-0.423832528941423,-0.12));
#65563=CARTESIAN_POINT('Origin',(0.,0.,-0.12));
#65564=CARTESIAN_POINT('Ctrl Pts',(0.11807574112921,-0.423808297522097,
-0.12));
#65565=CARTESIAN_POINT('Ctrl Pts',(0.125113297528677,-0.421379174521328,
-0.12));
#65566=CARTESIAN_POINT('Ctrl Pts',(0.132087840054081,-0.418769592094058,
-0.120000000000008));
#65567=CARTESIAN_POINT('Ctrl Pts',(0.145881768282444,-0.413195704088879,
-0.120000000000008));
#65568=CARTESIAN_POINT('Ctrl Pts',(0.15269989343557,-0.410232605099891,
-0.12));
#65569=CARTESIAN_POINT('Ctrl Pts',(0.159436307123189,-0.407092009220176,
-0.12));
#65570=CARTESIAN_POINT('Ctrl Pts',(-0.191616906624657,0.39225821899835,
-0.769079186525837));
#65571=CARTESIAN_POINT('Ctrl Pts',(-0.256609926003248,0.3605093333859,-0.766442158211432));
#65572=CARTESIAN_POINT('Ctrl Pts',(-0.36955373332459,0.26409422716641,-0.761168101582621));
#65573=CARTESIAN_POINT('Ctrl Pts',(-0.480807942249448,-0.0140930329678582,
-0.750619988324998));
#65574=CARTESIAN_POINT('Ctrl Pts',(-0.332057960250246,-0.3941381812961,
-0.737434846752968));
#65575=CARTESIAN_POINT('Ctrl Pts',(0.15018603425576,-0.493306196243262,
-0.721612676866535));
#65576=CARTESIAN_POINT('Ctrl Pts',(0.494996424724238,-0.143038083793679,
-0.705790506980099));
#65577=CARTESIAN_POINT('Ctrl Pts',(0.390010833532397,0.336947617464268,
-0.689968337093666));
#65578=CARTESIAN_POINT('Ctrl Pts',(-0.0699280367938378,0.510661735563277,
-0.674146167207231));
#65579=CARTESIAN_POINT('Ctrl Pts',(-0.466149582960942,0.219803044164238,
-0.658323997320798));
#65580=CARTESIAN_POINT('Ctrl Pts',(-0.438446333712939,-0.270923223572784,
-0.642501827434362));
#65581=CARTESIAN_POINT('Ctrl Pts',(-0.0119251715759321,-0.515260161789781,
-0.626679657547929));
#65582=CARTESIAN_POINT('Ctrl Pts',(0.425426395664575,-0.290930041698329,
-0.610857487661495));
#65583=CARTESIAN_POINT('Ctrl Pts',(0.475841582620101,0.198006753256743,
-0.59503531777506));
#65584=CARTESIAN_POINT('Ctrl Pts',(0.0934527706364431,0.506851252932052,
-0.579213147888625));
#65585=CARTESIAN_POINT('Ctrl Pts',(-0.373933347002199,0.354689364040992,
-0.563390978002191));
#65586=CARTESIAN_POINT('Ctrl Pts',(-0.501211178777902,-0.120077651523246,
-0.547568808115756));
#65587=CARTESIAN_POINT('Ctrl Pts',(-0.172613939570439,-0.485629104653691,
-0.531746638229323));
#65588=CARTESIAN_POINT('Ctrl Pts',(0.312983245232899,-0.409478420630284,
-0.515924468342887));
#65589=CARTESIAN_POINT('Ctrl Pts',(0.513908037004678,0.0391114426547363,
-0.500102298456454));
#65590=CARTESIAN_POINT('Ctrl Pts',(0.247409909573403,0.452127740210172,
-0.484280128570019));
#65591=CARTESIAN_POINT('Ctrl Pts',(-0.244118787161056,0.453913163939864,
-0.468457958683585));
#65592=CARTESIAN_POINT('Ctrl Pts',(-0.513610319356525,0.0428438566086168,
-0.45263578879715));
#65593=CARTESIAN_POINT('Ctrl Pts',(-0.31594979384439,-0.407193914453912,
-0.436813618910716));
#65594=CARTESIAN_POINT('Ctrl Pts',(0.169081494863269,-0.486870199065095,
-0.420991449024282));
#65595=CARTESIAN_POINT('Ctrl Pts',(0.500325443658047,-0.123715832661201,
-0.405169279137847));
#65596=CARTESIAN_POINT('Ctrl Pts',(0.376500546994966,0.35196379580438,-0.389347109251413));
#65597=CARTESIAN_POINT('Ctrl Pts',(-0.0897687952733545,0.50751615949993,
-0.373524939364978));
#65598=CARTESIAN_POINT('Ctrl Pts',(-0.474389315494283,0.201459615718978,
-0.357702769478544));
#65599=CARTESIAN_POINT('Ctrl Pts',(-0.427531089604827,-0.287834076420048,
-0.34188059959211));
#65600=CARTESIAN_POINT('Ctrl Pts',(0.0081862010117207,-0.515328709734928,
-0.326058429705676));
#65601=CARTESIAN_POINT('Ctrl Pts',(0.43645774796877,-0.274109918055601,
-0.310236259819241));
#65602=CARTESIAN_POINT('Ctrl Pts',(0.467751075340982,0.216427395685096,
-0.294414089932807));
#65603=CARTESIAN_POINT('Ctrl Pts',(0.0736033601307095,0.510108275435923,
-0.278591920046372));
#65604=CARTESIAN_POINT('Ctrl Pts',(-0.387489830816053,0.339833599072979,
-0.262769750159938));
#65605=CARTESIAN_POINT('Ctrl Pts',(-0.49614359495678,-0.139556847917794,
-0.246947580273503));
#65606=CARTESIAN_POINT('Ctrl Pts',(-0.153531570178307,-0.491972426948004,
-0.231125410387069));
#65607=CARTESIAN_POINT('Ctrl Pts',(0.328723417402025,-0.396996540727841,
-0.215303240500635));
#65608=CARTESIAN_POINT('Ctrl Pts',(0.511991387155289,0.0592196476372865,
-0.199481070614201));
#65609=CARTESIAN_POINT('Ctrl Pts',(0.229576097471973,0.461276673347663,
-0.183658900727766));
#65610=CARTESIAN_POINT('Ctrl Pts',(-0.261642352685609,0.444353606285138,
-0.167836730841332));
#65611=CARTESIAN_POINT('Ctrl Pts',(-0.514894954705951,0.0221490527857774,
-0.152014560954898));
#65612=CARTESIAN_POINT('Ctrl Pts',(-0.335682896194775,-0.344516885087901,
-0.138829419382869));
#65613=CARTESIAN_POINT('Ctrl Pts',(-0.0554577497370425,-0.450848389249885,
-0.128277377956503));
#65614=CARTESIAN_POINT('Ctrl Pts',(0.0920701638712636,-0.432846326389371,
-0.122999393158948));
#65615=CARTESIAN_POINT('Ctrl Pts',(0.159503405388502,-0.406376930613758,
-0.120358436675798));
#65616=CARTESIAN_POINT('Ctrl Pts',(-0.200102980078069,0.409630026725342,
-0.757916851848296));
#65617=CARTESIAN_POINT('Ctrl Pts',(-0.267974323431935,0.376475088901128,
-0.755279823533891));
#65618=CARTESIAN_POINT('Ctrl Pts',(-0.385920035135933,0.275790079321805,
-0.750005766905079));
#65619=CARTESIAN_POINT('Ctrl Pts',(-0.502101321767911,-0.0147171663757771,
-0.739457653647457));
#65620=CARTESIAN_POINT('Ctrl Pts',(-0.346763699378963,-0.411593246280656,
-0.726272512075427));
#65621=CARTESIAN_POINT('Ctrl Pts',(0.156837272608476,-0.515153081729957,
-0.710450342188994));
#65622=CARTESIAN_POINT('Ctrl Pts',(0.51691816479081,-0.149372763269987,
-0.694628172302559));
#65623=CARTESIAN_POINT('Ctrl Pts',(0.407283112055635,0.351869903196366,
-0.678806002416125));
#65624=CARTESIAN_POINT('Ctrl Pts',(-0.0730249162244601,0.533277239978685,
-0.66298383252969));
#65625=CARTESIAN_POINT('Ctrl Pts',(-0.486793792654988,0.229537387604584,
-0.647161662643257));
#65626=CARTESIAN_POINT('Ctrl Pts',(-0.457863658931299,-0.282921509193673,
-0.631339492756821));
#65627=CARTESIAN_POINT('Ctrl Pts',(-0.0124532976359992,-0.538079315159844,
-0.615517322870387));
#65628=CARTESIAN_POINT('Ctrl Pts',(0.444267111268556,-0.303814362540081,
-0.599695152983953));
#65629=CARTESIAN_POINT('Ctrl Pts',(0.496915018641129,0.206775811697394,
-0.583872983097518));
#65630=CARTESIAN_POINT('Ctrl Pts',(0.097591482037307,0.529298003785622,
-0.568050813211084));
#65631=CARTESIAN_POINT('Ctrl Pts',(-0.390493607290488,0.3703973725326,-0.55222864332465));
#65632=CARTESIAN_POINT('Ctrl Pts',(-0.52340814956562,-0.125395490063117,
-0.536406473438216));
#65633=CARTESIAN_POINT('Ctrl Pts',(-0.180258435017528,-0.507135997368949,
-0.520584303551781));
#65634=CARTESIAN_POINT('Ctrl Pts',(0.326844228877396,-0.427612853631347,
-0.504762133665347));
#65635=CARTESIAN_POINT('Ctrl Pts',(0.536667309279451,0.0408435579523025,
-0.488939963778913));
#65636=CARTESIAN_POINT('Ctrl Pts',(0.258366868970805,0.472150969273484,
-0.473117793892478));
#65637=CARTESIAN_POINT('Ctrl Pts',(-0.254929993727836,0.474015463462993,
-0.457295624006044));
#65638=CARTESIAN_POINT('Ctrl Pts',(-0.536356406710014,0.0447412680667841,
-0.441473454119609));
#65639=CARTESIAN_POINT('Ctrl Pts',(-0.329942156028828,-0.425227174298811,
-0.425651284233175));
#65640=CARTESIAN_POINT('Ctrl Pts',(0.176569550120485,-0.508432055710849,
-0.409829114346741));
#65641=CARTESIAN_POINT('Ctrl Pts',(0.522483188192614,-0.129194794104669,
-0.394006944460306));
#65642=CARTESIAN_POINT('Ctrl Pts',(0.39317450000532,0.367551097972806,-0.378184774573872));
#65643=CARTESIAN_POINT('Ctrl Pts',(-0.093744355697186,0.529992356846891,
-0.362362604687438));
#65644=CARTESIAN_POINT('Ctrl Pts',(-0.495398435449882,0.210381589917405,
-0.346540434801003));
#65645=CARTESIAN_POINT('Ctrl Pts',(-0.446465015080988,-0.300581287289494,
-0.330718264914569));
#65646=CARTESIAN_POINT('Ctrl Pts',(0.00854874054079198,-0.538150898864768,
-0.314896095028135));
#65647=CARTESIAN_POINT('Ctrl Pts',(0.455787005359554,-0.286249331742543,
-0.299073925141701));
#65648=CARTESIAN_POINT('Ctrl Pts',(0.488466209789068,0.22601224291735,-0.283251755255266));
#65649=CARTESIAN_POINT('Ctrl Pts',(0.0768630073689911,0.532699268948942,
-0.267429585368832));
#65650=CARTESIAN_POINT('Ctrl Pts',(-0.404650462540456,0.354883695301281,
-0.251607415482397));
#65651=CARTESIAN_POINT('Ctrl Pts',(-0.51811613936535,-0.145737355072503,
-0.235785245595963));
#65652=CARTESIAN_POINT('Ctrl Pts',(-0.160330971154458,-0.513760244242811,
-0.219963075709529));
#65653=CARTESIAN_POINT('Ctrl Pts',(0.343281480753889,-0.414578192914544,
-0.204140905823094));
#65654=CARTESIAN_POINT('Ctrl Pts',(0.534665777403248,0.0618422882413304,
-0.18831873593666));
#65655=CARTESIAN_POINT('Ctrl Pts',(0.239743256834957,0.481705078133685,
-0.172496566050225));
#65656=CARTESIAN_POINT('Ctrl Pts',(-0.273229619501072,0.464032544895762,
-0.156674396163791));
#65657=CARTESIAN_POINT('Ctrl Pts',(-0.537697934272806,0.0231299604320526,
-0.140852226277357));
#65658=CARTESIAN_POINT('Ctrl Pts',(-0.350549171641664,-0.359774388427747,
-0.127667084705328));
#65659=CARTESIAN_POINT('Ctrl Pts',(-0.0579137884348772,-0.470814960127794,
-0.117115043278961));
#65660=CARTESIAN_POINT('Ctrl Pts',(0.0961476442316455,-0.452015645968122,
-0.111837058481407));
#65661=CARTESIAN_POINT('Ctrl Pts',(0.166567279020736,-0.424374008970292,
-0.109196101998257));
#65662=CARTESIAN_POINT('Ctrl Pts',(-0.208589053531481,0.427001834452336,
-0.746754517170756));
#65663=CARTESIAN_POINT('Ctrl Pts',(-0.279338720860621,0.392440844416355,
-0.74411748885635));
#65664=CARTESIAN_POINT('Ctrl Pts',(-0.402286336947276,0.287485931477201,
-0.738843432227539));
#65665=CARTESIAN_POINT('Ctrl Pts',(-0.523394701286374,-0.0153412997836962,
-0.728295318969915));
#65666=CARTESIAN_POINT('Ctrl Pts',(-0.361469438507679,-0.429048311265211,
-0.715110177397887));
#65667=CARTESIAN_POINT('Ctrl Pts',(0.163488510961194,-0.536999967216652,
-0.699288007511452));
#65668=CARTESIAN_POINT('Ctrl Pts',(0.538839904857383,-0.155707442746293,
-0.683465837625019));
#65669=CARTESIAN_POINT('Ctrl Pts',(0.424555390578873,0.366792188928465,
-0.667643667738583));
#65670=CARTESIAN_POINT('Ctrl Pts',(-0.076121795655082,0.555892744394093,
-0.65182149785215));
#65671=CARTESIAN_POINT('Ctrl Pts',(-0.507438002349034,0.239271731044931,
-0.635999327965715));
#65672=CARTESIAN_POINT('Ctrl Pts',(-0.47728098414966,-0.294919794814562,
-0.620177158079281));
#65673=CARTESIAN_POINT('Ctrl Pts',(-0.0129814236960666,-0.560898468529907,
-0.604354988192846));
#65674=CARTESIAN_POINT('Ctrl Pts',(0.463107826872538,-0.316698683381835,
-0.588532818306413));
#65675=CARTESIAN_POINT('Ctrl Pts',(0.517988454662157,0.215544870138044,
-0.572710648419977));
#65676=CARTESIAN_POINT('Ctrl Pts',(0.101730193438172,0.551744754639191,
-0.556888478533544));
#65677=CARTESIAN_POINT('Ctrl Pts',(-0.407053867578776,0.386105381024208,
-0.541066308647109));
#65678=CARTESIAN_POINT('Ctrl Pts',(-0.545605120353339,-0.130713328602987,
-0.525244138760675));
#65679=CARTESIAN_POINT('Ctrl Pts',(-0.187902930464619,-0.528642890084206,
-0.50942196887424));
#65680=CARTESIAN_POINT('Ctrl Pts',(0.340705212521894,-0.445747286632409,
-0.493599798987806));
#65681=CARTESIAN_POINT('Ctrl Pts',(0.559426581554225,0.042575673249869,
-0.477777629101371));
#65682=CARTESIAN_POINT('Ctrl Pts',(0.269323828368205,0.492174198336795,
-0.461955459214937));
#65683=CARTESIAN_POINT('Ctrl Pts',(-0.265741200294616,0.494117762986121,
-0.446133289328503));
#65684=CARTESIAN_POINT('Ctrl Pts',(-0.559102494063503,0.0466386795249515,
-0.430311119442069));
#65685=CARTESIAN_POINT('Ctrl Pts',(-0.343934518213266,-0.44326043414371,
-0.414488949555634));
#65686=CARTESIAN_POINT('Ctrl Pts',(0.184057605377702,-0.529993912356603,
-0.3986667796692));
#65687=CARTESIAN_POINT('Ctrl Pts',(0.544640932727182,-0.134673755548136,
-0.382844609782765));
#65688=CARTESIAN_POINT('Ctrl Pts',(0.409848453015675,0.383138400141232,
-0.367022439896332));
#65689=CARTESIAN_POINT('Ctrl Pts',(-0.097719916121017,0.552468554193852,
-0.351200270009897));
#65690=CARTESIAN_POINT('Ctrl Pts',(-0.516407555405482,0.219303564115831,
-0.335378100123463));
#65691=CARTESIAN_POINT('Ctrl Pts',(-0.46539894055715,-0.31332849815894,
-0.319555930237028));
#65692=CARTESIAN_POINT('Ctrl Pts',(0.00891128006986319,-0.560973087994608,
-0.303733760350594));
#65693=CARTESIAN_POINT('Ctrl Pts',(0.475116262750338,-0.298388745429484,
-0.287911590464159));
#65694=CARTESIAN_POINT('Ctrl Pts',(0.509181344237154,0.235597090149604,
-0.272089420577725));
#65695=CARTESIAN_POINT('Ctrl Pts',(0.0801226546072732,0.555290262461962,
-0.25626725069129));
#65696=CARTESIAN_POINT('Ctrl Pts',(-0.421811094264861,0.369933791529583,
-0.240445080804857));
#65697=CARTESIAN_POINT('Ctrl Pts',(-0.54008868377392,-0.151917862227212,
-0.224622910918422));
#65698=CARTESIAN_POINT('Ctrl Pts',(-0.16713037213061,-0.535548061537618,
-0.208800741031988));
#65699=CARTESIAN_POINT('Ctrl Pts',(0.357839544105755,-0.43215984510125,
-0.192978571145553));
#65700=CARTESIAN_POINT('Ctrl Pts',(0.557340167651207,0.0644649288453748,
-0.177156401259119));
#65701=CARTESIAN_POINT('Ctrl Pts',(0.249910416197941,0.502133482919706,
-0.161334231372684));
#65702=CARTESIAN_POINT('Ctrl Pts',(-0.284816886316535,0.483711483506385,
-0.14551206148625));
#65703=CARTESIAN_POINT('Ctrl Pts',(-0.560500913839662,0.0241108680783272,
-0.129689891599816));
#65704=CARTESIAN_POINT('Ctrl Pts',(-0.365415447088553,-0.375031891767592,
-0.116504750027787));
#65705=CARTESIAN_POINT('Ctrl Pts',(-0.0603698271327118,-0.490781531005703,
-0.10595270860142));
#65706=CARTESIAN_POINT('Ctrl Pts',(0.100225124592028,-0.471184965546873,
-0.100674723803866));
#65707=CARTESIAN_POINT('Ctrl Pts',(0.17363115265297,-0.442371087326825,
-0.098033767320716));
#65708=CARTESIAN_POINT('Ctrl Pts',(-0.217075126984893,0.444373642179328,
-0.735592182493215));
#65709=CARTESIAN_POINT('Ctrl Pts',(-0.290703118289308,0.408406599931581,
-0.732955154178809));
#65710=CARTESIAN_POINT('Ctrl Pts',(-0.418652638758619,0.299181783632597,
-0.727681097549997));
#65711=CARTESIAN_POINT('Ctrl Pts',(-0.544688080804837,-0.0159654331916153,
-0.717132984292375));
#65712=CARTESIAN_POINT('Ctrl Pts',(-0.376175177636396,-0.446503376249768,
-0.703947842720345));
#65713=CARTESIAN_POINT('Ctrl Pts',(0.170139749313912,-0.558846852703347,
-0.688125672833912));
#65714=CARTESIAN_POINT('Ctrl Pts',(0.560761644923954,-0.162042122222599,
-0.672303502947477));
#65715=CARTESIAN_POINT('Ctrl Pts',(0.441827669102111,0.381714474660563,
-0.656481333061043));
#65716=CARTESIAN_POINT('Ctrl Pts',(-0.0792186750857043,0.578508248809501,
-0.640659163174609));
#65717=CARTESIAN_POINT('Ctrl Pts',(-0.528082212043081,0.249006074485278,
-0.624836993288174));
#65718=CARTESIAN_POINT('Ctrl Pts',(-0.496698309368021,-0.30691808043545,
-0.60901482340174));
#65719=CARTESIAN_POINT('Ctrl Pts',(-0.0135095497561338,-0.58371762189997,
-0.593192653515305));
#65720=CARTESIAN_POINT('Ctrl Pts',(0.48194854247652,-0.329583004223587,
-0.577370483628871));
#65721=CARTESIAN_POINT('Ctrl Pts',(0.539061890683185,0.224313928578695,
-0.561548313742437));
#65722=CARTESIAN_POINT('Ctrl Pts',(0.105868904839035,0.57419150549276,-0.545726143856003));
#65723=CARTESIAN_POINT('Ctrl Pts',(-0.423614127867063,0.401813389515817,
-0.529903973969568));
#65724=CARTESIAN_POINT('Ctrl Pts',(-0.567802091141058,-0.136031167142859,
-0.514081804083134));
#65725=CARTESIAN_POINT('Ctrl Pts',(-0.195547425911708,-0.550149782799461,
-0.498259634196699));
#65726=CARTESIAN_POINT('Ctrl Pts',(0.354566196166392,-0.463881719633473,
-0.482437464310265));
#65727=CARTESIAN_POINT('Ctrl Pts',(0.582185853828999,0.044307788547436,
-0.466615294423831));
#65728=CARTESIAN_POINT('Ctrl Pts',(0.280280787765607,0.512197427400107,
-0.450793124537396));
#65729=CARTESIAN_POINT('Ctrl Pts',(-0.276552406861396,0.514220062509251,
-0.434970954650963));
#65730=CARTESIAN_POINT('Ctrl Pts',(-0.581848581416993,0.0485360909831188,
-0.419148784764527));
#65731=CARTESIAN_POINT('Ctrl Pts',(-0.357926880397705,-0.461293693988608,
-0.403326614878094));
#65732=CARTESIAN_POINT('Ctrl Pts',(0.191545660634918,-0.551555769002358,
-0.387504444991659));
#65733=CARTESIAN_POINT('Ctrl Pts',(0.566798677261749,-0.140152716991604,
-0.371682275105225));
#65734=CARTESIAN_POINT('Ctrl Pts',(0.42652240602603,0.398725702309659,-0.35586010521879));
#65735=CARTESIAN_POINT('Ctrl Pts',(-0.101695476544849,0.574944751540813,
-0.340037935332356));
#65736=CARTESIAN_POINT('Ctrl Pts',(-0.537416675361082,0.228225538314257,
-0.324215765445922));
#65737=CARTESIAN_POINT('Ctrl Pts',(-0.484332866033311,-0.326075709028386,
-0.308393595559487));
#65738=CARTESIAN_POINT('Ctrl Pts',(0.00927381959893476,-0.583795277124447,
-0.292571425673053));
#65739=CARTESIAN_POINT('Ctrl Pts',(0.494445520141122,-0.310528159116424,
-0.276749255786619));
#65740=CARTESIAN_POINT('Ctrl Pts',(0.52989647868524,0.245181937381857,-0.260927085900184));
#65741=CARTESIAN_POINT('Ctrl Pts',(0.083382301845555,0.577881255974982,
-0.24510491601375));
#65742=CARTESIAN_POINT('Ctrl Pts',(-0.438971725989264,0.384983887757886,
-0.229282746127315));
#65743=CARTESIAN_POINT('Ctrl Pts',(-0.562061228182491,-0.158098369381922,
-0.213460576240881));
#65744=CARTESIAN_POINT('Ctrl Pts',(-0.173929773106761,-0.557335878832425,
-0.197638406354447));
#65745=CARTESIAN_POINT('Ctrl Pts',(0.37239760745762,-0.449741497287954,
-0.181816236468012));
#65746=CARTESIAN_POINT('Ctrl Pts',(0.580014557899165,0.0670875694494189,
-0.165994066581578));
#65747=CARTESIAN_POINT('Ctrl Pts',(0.260077575560924,0.522561887705728,
-0.150171896695144));
#65748=CARTESIAN_POINT('Ctrl Pts',(-0.296404153131998,0.503390422117009,
-0.134349726808709));
#65749=CARTESIAN_POINT('Ctrl Pts',(-0.583303893406517,0.0250917757246023,
-0.118527556922275));
#65750=CARTESIAN_POINT('Ctrl Pts',(-0.380281722535441,-0.390289395107438,
-0.105342415350246));
#65751=CARTESIAN_POINT('Ctrl Pts',(-0.0628258658305463,-0.510748101883613,
-0.0947903739238797));
#65752=CARTESIAN_POINT('Ctrl Pts',(0.104302604952409,-0.490354285125624,
-0.0895123891263246));
#65753=CARTESIAN_POINT('Ctrl Pts',(0.180695026285204,-0.460368165683359,
-0.0868714326431751));
#65754=CARTESIAN_POINT('',(0.117283993805721,-0.424080729103529,-0.119999999999908));
#65755=CARTESIAN_POINT('Ctrl Pts',(0.117283993805721,-0.424080729103529,
-0.12));
#65756=CARTESIAN_POINT('Ctrl Pts',(0.117550426203052,-0.423997995716161,
-0.12));
#65757=CARTESIAN_POINT('Ctrl Pts',(0.117816858600383,-0.423915262328792,
-0.12));
#65758=CARTESIAN_POINT('Ctrl Pts',(0.118083290997715,-0.423832528941423,
-0.12));
#65759=CARTESIAN_POINT('Ctrl Pts',(-0.491123371243679,0.0606208880126489,
-0.12));
#65760=CARTESIAN_POINT('Ctrl Pts',(-0.492080117217891,0.047615190510706,
-0.12));
#65761=CARTESIAN_POINT('Ctrl Pts',(-0.492488068218865,0.0346059367317309,
-0.12));
#65762=CARTESIAN_POINT('Ctrl Pts',(-0.492330824576398,0.0216199151589219,
-0.119999999999999));
#65763=CARTESIAN_POINT('Ctrl Pts',(-0.49201965108577,-0.00407845711732452,
-0.119999999999999));
#65764=CARTESIAN_POINT('Ctrl Pts',(-0.489498465803643,-0.0296866016555778,
-0.119999999999999));
#65765=CARTESIAN_POINT('Ctrl Pts',(-0.484915318387734,-0.054991083609342,
-0.119999999999999));
#65766=CARTESIAN_POINT('Ctrl Pts',(-0.481966249957855,-0.0712734856558606,
-0.119999999999999));
#65767=CARTESIAN_POINT('Ctrl Pts',(-0.478162287482436,-0.0874300941371983,
-0.119999999999999));
#65768=CARTESIAN_POINT('Ctrl Pts',(-0.47353228316563,-0.10340020940642,
-0.119999999999999));
#65769=CARTESIAN_POINT('Ctrl Pts',(-0.471503718009439,-0.110397269702435,
-0.119999999999999));
#65770=CARTESIAN_POINT('Ctrl Pts',(-0.469316487641571,-0.117358474639077,
-0.119999999999999));
#65771=CARTESIAN_POINT('Ctrl Pts',(-0.466972594711345,-0.124278411688063,
-0.119999999999999));
#65772=CARTESIAN_POINT('Ctrl Pts',(-0.464920047601107,-0.130338200772182,
-0.119999999999999));
#65773=CARTESIAN_POINT('Ctrl Pts',(-0.462750029372983,-0.136358237212316,
-0.119999999999999));
#65774=CARTESIAN_POINT('Ctrl Pts',(-0.460466874239735,-0.142329905900782,
-0.119999999999999));
#65775=CARTESIAN_POINT('Ctrl Pts',(-0.454534266424897,-0.157846840257503,
-0.119999999999998));
#65776=CARTESIAN_POINT('Ctrl Pts',(-0.447834494625283,-0.173049044034483,
-0.119999999999999));
#65777=CARTESIAN_POINT('Ctrl Pts',(-0.440405049160724,-0.187879519724027,
-0.119999999999999));
#65778=CARTESIAN_POINT('Ctrl Pts',(-0.430752165148136,-0.207148368572245,
-0.119999999999998));
#65779=CARTESIAN_POINT('Ctrl Pts',(-0.419868031369589,-0.225790477133216,
-0.119999999999999));
#65780=CARTESIAN_POINT('Ctrl Pts',(-0.407815725943723,-0.243668211022738,
-0.119999999999999));
#65781=CARTESIAN_POINT('Ctrl Pts',(-0.401748202520733,-0.252668445027085,
-0.119999999999999));
#65782=CARTESIAN_POINT('Ctrl Pts',(-0.395384296714486,-0.261474691340732,
-0.119999999999999));
#65783=CARTESIAN_POINT('Ctrl Pts',(-0.388730354116756,-0.27006745480899,
-0.119999999999999));
#65784=CARTESIAN_POINT('Ctrl Pts',(-0.383733104832073,-0.27652079889252,
-0.119999999999999));
#65785=CARTESIAN_POINT('Ctrl Pts',(-0.378570178487854,-0.282856065934985,
-0.119999999999999));
#65786=CARTESIAN_POINT('Ctrl Pts',(-0.373251230417089,-0.289056005825397,
-0.119999999999999));
#65787=CARTESIAN_POINT('Ctrl Pts',(-0.366987352291694,-0.296357387102605,
-0.119999999999999));
#65788=CARTESIAN_POINT('Ctrl Pts',(-0.360518140092558,-0.303458590347285,
-0.119999999999999));
#65789=CARTESIAN_POINT('Ctrl Pts',(-0.353851489645469,-0.31034682109201,
-0.119999999999999));
#65790=CARTESIAN_POINT('Ctrl Pts',(-0.336767631137862,-0.327998497949016,
-0.119999999999999));
#65791=CARTESIAN_POINT('Ctrl Pts',(-0.318385138846978,-0.344259173584621,
-0.119999999999999));
#65792=CARTESIAN_POINT('Ctrl Pts',(-0.298792194188593,-0.35891278731163,
-0.119999999999999));
#65793=CARTESIAN_POINT('Ctrl Pts',(-0.289653252506453,-0.365747825312231,
-0.119999999999999));
#65794=CARTESIAN_POINT('Ctrl Pts',(-0.280250534791944,-0.37223265094451,
-0.119999999999999));
#65795=CARTESIAN_POINT('Ctrl Pts',(-0.270591090586766,-0.378341879595979,
-0.119999999999999));
#65796=CARTESIAN_POINT('Ctrl Pts',(-0.260227879567575,-0.384896213813854,
-0.12));
#65797=CARTESIAN_POINT('Ctrl Pts',(-0.249569109631511,-0.391018236754718,
-0.119999999999999));
#65798=CARTESIAN_POINT('Ctrl Pts',(-0.23864629776066,-0.396699229261459,
-0.12));
#65799=CARTESIAN_POINT('Ctrl Pts',(-0.232340801497141,-0.399978739835099,
-0.12));
#65800=CARTESIAN_POINT('Ctrl Pts',(-0.225949975898595,-0.403109514421454,
-0.12));
#65801=CARTESIAN_POINT('Ctrl Pts',(-0.219496623082571,-0.406083117869338,
-0.12));
#65802=CARTESIAN_POINT('Ctrl Pts',(-0.197213019410682,-0.416351051856378,
-0.12));
#65803=CARTESIAN_POINT('Ctrl Pts',(-0.174132212877899,-0.424776976216567,
-0.12));
#65804=CARTESIAN_POINT('Ctrl Pts',(-0.150520658792025,-0.431330470391991,
-0.12));
#65805=CARTESIAN_POINT('Ctrl Pts',(-0.135040134457732,-0.435627160295939,
-0.12));
#65806=CARTESIAN_POINT('Ctrl Pts',(-0.119330949077229,-0.439117977054067,
-0.12));
#65807=CARTESIAN_POINT('Ctrl Pts',(-0.103466627673514,-0.441782460714082,
-0.12));
#65808=CARTESIAN_POINT('Ctrl Pts',(-0.0936646074926034,-0.443428753797949,
-0.12));
#65809=CARTESIAN_POINT('Ctrl Pts',(-0.0838033584053894,-0.444759400455696,
-0.12));
#65810=CARTESIAN_POINT('Ctrl Pts',(-0.0739005440596103,-0.44576771286662,
-0.12));
#65811=CARTESIAN_POINT('Ctrl Pts',(-0.067775904198683,-0.446391328554906,
-0.12));
#65812=CARTESIAN_POINT('Ctrl Pts',(-0.0616324034529957,-0.446891719509591,
-0.12));
#65813=CARTESIAN_POINT('Ctrl Pts',(-0.0554891763724216,-0.447266361985043,
-0.12));
#65814=CARTESIAN_POINT('Ctrl Pts',(-0.0312303804256718,-0.448745775857556,
-0.12));
#65815=CARTESIAN_POINT('Ctrl Pts',(-0.00694611010869578,-0.448273303612837,
-0.120000000000001));
#65816=CARTESIAN_POINT('Ctrl Pts',(0.0171508719125321,-0.445867538950042,
-0.12));
#65817=CARTESIAN_POINT('Ctrl Pts',(0.0278703336077171,-0.444797342602311,
-0.12));
#65818=CARTESIAN_POINT('Ctrl Pts',(0.0385536205803394,-0.443343713284888,
-0.120000000000001));
#65819=CARTESIAN_POINT('Ctrl Pts',(0.0491779042183454,-0.441505648869441,
-0.12));
#65820=CARTESIAN_POINT('Ctrl Pts',(0.0567863132575334,-0.440189348741395,
-0.12));
#65821=CARTESIAN_POINT('Ctrl Pts',(0.0643592452838578,-0.438676618147634,
-0.119999999999995));
#65822=CARTESIAN_POINT('Ctrl Pts',(0.0718799379532853,-0.436969919520122,
-0.119999999999986));
#65823=CARTESIAN_POINT('Ctrl Pts',(0.0872391156201996,-0.433484404475689,
-0.119999999999966));
#65824=CARTESIAN_POINT('Ctrl Pts',(0.102394078399616,-0.42918816774082,
-0.11999999999993));
#65825=CARTESIAN_POINT('Ctrl Pts',(0.117283993805721,-0.424080729103529,
-0.119999999999908));
#65826=CARTESIAN_POINT('Ctrl Pts',(-0.254468725618617,-0.356220527001759,
-0.735799999999999));
#65827=CARTESIAN_POINT('Ctrl Pts',(-0.264353107583362,-0.350156188421938,
-0.7358));
#65828=CARTESIAN_POINT('Ctrl Pts',(-0.273959725733427,-0.343690194162452,
-0.7358));
#65829=CARTESIAN_POINT('Ctrl Pts',(-0.283259413984319,-0.33682783052223,
-0.7358));
#65830=CARTESIAN_POINT('Ctrl Pts',(-0.298891697970022,-0.32529256026983,
-0.7358));
#65831=CARTESIAN_POINT('Ctrl Pts',(-0.313657637511065,-0.312638532827742,
-0.7358));
#65832=CARTESIAN_POINT('Ctrl Pts',(-0.327524596172051,-0.299000188399973,
-0.7358));
#65833=CARTESIAN_POINT('Ctrl Pts',(-0.335926090867447,-0.290737202898599,
-0.7358));
#65834=CARTESIAN_POINT('Ctrl Pts',(-0.34400320179419,-0.28210496066844,
-0.7358));
#65835=CARTESIAN_POINT('Ctrl Pts',(-0.35171720368204,-0.27316538278638,
-0.7358));
#65836=CARTESIAN_POINT('Ctrl Pts',(-0.362858848127632,-0.260253589439211,
-0.7358));
#65837=CARTESIAN_POINT('Ctrl Pts',(-0.373251963872608,-0.246695048235492,
-0.7358));
#65838=CARTESIAN_POINT('Ctrl Pts',(-0.382874250241917,-0.232577275099803,
-0.7358));
#65839=CARTESIAN_POINT('Ctrl Pts',(-0.38925049206296,-0.223222083201244,
-0.7358));
#65840=CARTESIAN_POINT('Ctrl Pts',(-0.395288097963382,-0.213621077157663,
-0.7358));
#65841=CARTESIAN_POINT('Ctrl Pts',(-0.400978371636687,-0.203797431456546,
-0.7358));
#65842=CARTESIAN_POINT('Ctrl Pts',(-0.406284528499182,-0.194636922130562,
-0.7358));
#65843=CARTESIAN_POINT('Ctrl Pts',(-0.41129110449982,-0.185276541719071,
-0.7358));
#65844=CARTESIAN_POINT('Ctrl Pts',(-0.415971025607449,-0.17577527097872,
-0.7358));
#65845=CARTESIAN_POINT('Ctrl Pts',(-0.426946975539136,-0.153491674837857,
-0.735799999999999));
#65846=CARTESIAN_POINT('Ctrl Pts',(-0.436153495753634,-0.130397933826654,
-0.735799999999999));
#65847=CARTESIAN_POINT('Ctrl Pts',(-0.443515830646781,-0.106740513259217,
-0.735799999999999));
#65848=CARTESIAN_POINT('Ctrl Pts',(-0.448460962867434,-0.0908502998413962,
-0.735799999999999));
#65849=CARTESIAN_POINT('Ctrl Pts',(-0.452573339202578,-0.0747048900916328,
-0.735799999999999));
#65850=CARTESIAN_POINT('Ctrl Pts',(-0.455818868496034,-0.0583724448329422,
-0.7358));
#65851=CARTESIAN_POINT('Ctrl Pts',(-0.457715300061376,-0.048829050850876,
-0.7358));
#65852=CARTESIAN_POINT('Ctrl Pts',(-0.459315495404145,-0.0392223922419898,
-0.735799999999999));
#65853=CARTESIAN_POINT('Ctrl Pts',(-0.460611248197923,-0.0295634006085556,
-0.735799999999999));
#65854=CARTESIAN_POINT('Ctrl Pts',(-0.461670102536421,-0.0216703323893049,
-0.7358));
#65855=CARTESIAN_POINT('Ctrl Pts',(-0.462524716732938,-0.0137458036513584,
-0.7358));
#65856=CARTESIAN_POINT('Ctrl Pts',(-0.46316948393252,-0.00582069942906378,
-0.7358));
#65857=CARTESIAN_POINT('Ctrl Pts',(-0.464873163375957,0.0151199395478807,
-0.7358));
#65858=CARTESIAN_POINT('Ctrl Pts',(-0.465119446792888,0.0361029865051353,
-0.7358));
#65859=CARTESIAN_POINT('Ctrl Pts',(-0.463852359252848,0.0569912948890308,
-0.7358));
#65860=CARTESIAN_POINT('Ctrl Pts',(-0.462665925504757,0.0765500019428417,
-0.7358));
#65861=CARTESIAN_POINT('Ctrl Pts',(-0.460152673100683,0.0960261356778588,
-0.735799999999999));
#65862=CARTESIAN_POINT('Ctrl Pts',(-0.45638650963416,0.11531015705626,-0.7358));
#65863=CARTESIAN_POINT('Ctrl Pts',(-0.454589389354817,0.124512016241201,
-0.7358));
#65864=CARTESIAN_POINT('Ctrl Pts',(-0.452506667493876,0.133670136132281,
-0.7358));
#65865=CARTESIAN_POINT('Ctrl Pts',(-0.450144715443353,0.142772427126565,
-0.7358));
#65866=CARTESIAN_POINT('Ctrl Pts',(-0.447579296485356,0.152658821675842,
-0.7358));
#65867=CARTESIAN_POINT('Ctrl Pts',(-0.444681359880229,0.162487158070278,
-0.7358));
#65868=CARTESIAN_POINT('Ctrl Pts',(-0.441474687718473,0.172195204108906,
-0.7358));
#65869=CARTESIAN_POINT('Ctrl Pts',(-0.433512738542325,0.19629962303926,
-0.7358));
#65870=CARTESIAN_POINT('Ctrl Pts',(-0.423642167106932,0.219710854775425,
-0.7358));
#65871=CARTESIAN_POINT('Ctrl Pts',(-0.412025148055811,0.242201623455124,
-0.7358));
#65872=CARTESIAN_POINT('Ctrl Pts',(-0.405546266354503,0.254744861010819,
-0.7358));
#65873=CARTESIAN_POINT('Ctrl Pts',(-0.398523189811845,0.267001785731961,
-0.7358));
#65874=CARTESIAN_POINT('Ctrl Pts',(-0.390977259868107,0.278931318470491,
-0.7358));
#65875=CARTESIAN_POINT('Ctrl Pts',(-0.383863888782996,0.290177009044596,
-0.7358));
#65876=CARTESIAN_POINT('Ctrl Pts',(-0.376285824866845,0.301131796958498,
-0.7358));
#65877=CARTESIAN_POINT('Ctrl Pts',(-0.368262330391237,0.311773139319828,
-0.7358));
#65878=CARTESIAN_POINT('Ctrl Pts',(-0.362781109777742,0.31904273304654,
-0.7358));
#65879=CARTESIAN_POINT('Ctrl Pts',(-0.35708820557215,0.326169789138345,
-0.7358));
#65880=CARTESIAN_POINT('Ctrl Pts',(-0.351214427199837,0.3331182156288,-0.735799999999999));
#65881=CARTESIAN_POINT('Ctrl Pts',(-0.334524773991188,0.352861355584183,
-0.735799999999999));
#65882=CARTESIAN_POINT('Ctrl Pts',(-0.316345467065958,0.371211611582931,
-0.735799999999999));
#65883=CARTESIAN_POINT('Ctrl Pts',(-0.296847946523699,0.388026973344292,
-0.735799999999999));
#65884=CARTESIAN_POINT('Ctrl Pts',(-0.277484732686358,0.404726504181137,
-0.735799999999999));
#65885=CARTESIAN_POINT('Ctrl Pts',(-0.256820572877241,0.419913180880695,
-0.7358));
#65886=CARTESIAN_POINT('Ctrl Pts',(-0.234984580042639,0.433415741977161,
-0.7358));
#65887=CARTESIAN_POINT('Ctrl Pts',(-0.229048153413863,0.437086606125949,
-0.7358));
#65888=CARTESIAN_POINT('Ctrl Pts',(-0.22302493302737,0.440632765949028,
-0.7358));
#65889=CARTESIAN_POINT('Ctrl Pts',(-0.21691713542861,0.4440502182833,-0.7358));
#65890=CARTESIAN_POINT('Origin',(-4.51336705371395E-17,0.,-0.7358));
#65891=CARTESIAN_POINT('',(-0.4942,-6.05220448138622E-17,-0.7358));
#65892=CARTESIAN_POINT('Origin',(0.,0.,-0.7358));
#65893=CARTESIAN_POINT('',(0.228820166259496,0.438035354181574,-0.7358));
#65894=CARTESIAN_POINT('Origin',(0.,0.,-0.7358));
#65895=CARTESIAN_POINT('Ctrl Pts',(0.228820166259493,0.438035354181575,
-0.735799999999999));
#65896=CARTESIAN_POINT('Ctrl Pts',(0.236316989062907,0.433616458939398,
-0.735799999999999));
#65897=CARTESIAN_POINT('Ctrl Pts',(0.243680112356663,0.428989449384103,
-0.735799999999998));
#65898=CARTESIAN_POINT('Ctrl Pts',(0.250899612637304,0.424153891241464,
-0.735799999999999));
#65899=CARTESIAN_POINT('Ctrl Pts',(0.267310017136389,0.413162345841524,
-0.735799999999999));
#65900=CARTESIAN_POINT('Ctrl Pts',(0.282979251405834,0.401094089156516,
-0.735799999999999));
#65901=CARTESIAN_POINT('Ctrl Pts',(0.297859083959773,0.388055028479292,
-0.735799999999999));
#65902=CARTESIAN_POINT('Ctrl Pts',(0.303851274087403,0.382804127275908,
-0.735799999999999));
#65903=CARTESIAN_POINT('Ctrl Pts',(0.309715294869631,0.377395648238053,
-0.735799999999999));
#65904=CARTESIAN_POINT('Ctrl Pts',(0.315447349016218,0.37183601851886,-0.735799999999999));
#65905=CARTESIAN_POINT('Ctrl Pts',(0.320512199566927,0.366923522418006,
-0.735799999999999));
#65906=CARTESIAN_POINT('Ctrl Pts',(0.325471210362565,0.361895553184773,
-0.735799999999999));
#65907=CARTESIAN_POINT('Ctrl Pts',(0.330316186686871,0.356763312701958,
-0.735799999999999));
#65908=CARTESIAN_POINT('Ctrl Pts',(0.347900557934295,0.338136344077132,
-0.735799999999999));
#65909=CARTESIAN_POINT('Ctrl Pts',(0.364009894806326,0.318115267361153,
-0.735799999999999));
#65910=CARTESIAN_POINT('Ctrl Pts',(0.378529988854265,0.296924385166985,
-0.735799999999999));
#65911=CARTESIAN_POINT('Ctrl Pts',(0.383986361678478,0.288961258113977,
-0.735799999999999));
#65912=CARTESIAN_POINT('Ctrl Pts',(0.389218397477593,0.280831801409261,
-0.735799999999999));
#65913=CARTESIAN_POINT('Ctrl Pts',(0.394216643597978,0.272550027802377,
-0.735799999999999));
#65914=CARTESIAN_POINT('Ctrl Pts',(0.398123146411223,0.266077202912462,
-0.7358));
#65915=CARTESIAN_POINT('Ctrl Pts',(0.40188294746496,0.259517556378562,-0.735799999999999));
#65916=CARTESIAN_POINT('Ctrl Pts',(0.405489037713727,0.252884933996346,
-0.735799999999999));
#65917=CARTESIAN_POINT('Ctrl Pts',(0.417666248863211,0.23048759015542,-0.735799999999999));
#65918=CARTESIAN_POINT('Ctrl Pts',(0.428112091848353,0.207230094193275,
-0.7358));
#65919=CARTESIAN_POINT('Ctrl Pts',(0.436709111403403,0.183328936062516,
-0.7358));
#65920=CARTESIAN_POINT('Ctrl Pts',(0.442380018901443,0.167562860856144,
-0.7358));
#65921=CARTESIAN_POINT('Ctrl Pts',(0.447245552684248,0.151516184828499,
-0.7358));
#65922=CARTESIAN_POINT('Ctrl Pts',(0.451259697186057,0.135248728490274,
-0.7358));
#65923=CARTESIAN_POINT('Ctrl Pts',(0.45361287992984,0.125712375844498,-0.7358));
#65924=CARTESIAN_POINT('Ctrl Pts',(0.455673284346557,0.116100135704311,
-0.7358));
#65925=CARTESIAN_POINT('Ctrl Pts',(0.457429894614468,0.106424173228407,
-0.7358));
#65926=CARTESIAN_POINT('Ctrl Pts',(0.45881226543766,0.0988096394542803,
-0.735799999999999));
#65927=CARTESIAN_POINT('Ctrl Pts',(0.460006040688075,0.0911556810687175,
-0.7358));
#65928=CARTESIAN_POINT('Ctrl Pts',(0.461003311645071,0.0834930990972771,
-0.7358));
#65929=CARTESIAN_POINT('Ctrl Pts',(0.46375279125733,0.0623673330655312,
-0.7358));
#65930=CARTESIAN_POINT('Ctrl Pts',(0.465020086686708,0.0411290663620106,
-0.7358));
#65931=CARTESIAN_POINT('Ctrl Pts',(0.464720781957338,0.0199037385120108,
-0.7358));
#65932=CARTESIAN_POINT('Ctrl Pts',(0.464453659527758,0.000960632748610985,
-0.7358));
#65933=CARTESIAN_POINT('Ctrl Pts',(0.462938198968576,-0.017972555627716,
-0.7358));
#65934=CARTESIAN_POINT('Ctrl Pts',(0.460221890912084,-0.0367828973530338,
-0.7358));
#65935=CARTESIAN_POINT('Ctrl Pts',(0.458149135112,-0.0511366613966768,-0.7358));
#65936=CARTESIAN_POINT('Ctrl Pts',(0.455376742418919,-0.0654188854679344,
-0.7358));
#65937=CARTESIAN_POINT('Ctrl Pts',(0.451919535610315,-0.0795763120724046,
-0.7358));
#65938=CARTESIAN_POINT('Ctrl Pts',(0.447468037670369,-0.0978054082340508,
-0.7358));
#65939=CARTESIAN_POINT('Ctrl Pts',(0.441907724804691,-0.115721130446471,
-0.7358));
#65940=CARTESIAN_POINT('Ctrl Pts',(0.435296532066892,-0.133213011861257,
-0.7358));
#65941=CARTESIAN_POINT('Ctrl Pts',(0.426856194344684,-0.155544441664159,
-0.7358));
#65942=CARTESIAN_POINT('Ctrl Pts',(0.416703258734146,-0.177189395420981,
-0.7358));
#65943=CARTESIAN_POINT('Ctrl Pts',(0.404917880756747,-0.19791002689791,
-0.7358));
#65944=CARTESIAN_POINT('Ctrl Pts',(0.398500717044332,-0.209192455401017,
-0.7358));
#65945=CARTESIAN_POINT('Ctrl Pts',(0.391598855565479,-0.220200352930322,
-0.7358));
#65946=CARTESIAN_POINT('Ctrl Pts',(0.384228438675215,-0.230904646838916,
-0.7358));
#65947=CARTESIAN_POINT('Ctrl Pts',(0.379522006890116,-0.237739949351449,
-0.7358));
#65948=CARTESIAN_POINT('Ctrl Pts',(0.374622283186425,-0.244453507108068,
-0.735799999999999));
#65949=CARTESIAN_POINT('Ctrl Pts',(0.369553954994059,-0.251011959085564,
-0.735799999999999));
#65950=CARTESIAN_POINT('Ctrl Pts',(0.354874618110099,-0.270007123242443,
-0.735799999999999));
#65951=CARTESIAN_POINT('Ctrl Pts',(0.338750738128904,-0.287754783607563,
-0.735799999999999));
#65952=CARTESIAN_POINT('Ctrl Pts',(0.321310977016985,-0.30409383577115,
-0.7358));
#65953=CARTESIAN_POINT('Ctrl Pts',(0.304262041952272,-0.32006672883822,
-0.7358));
#65954=CARTESIAN_POINT('Ctrl Pts',(0.285954603339099,-0.334694148798622,
-0.7358));
#65955=CARTESIAN_POINT('Ctrl Pts',(0.26648175861671,-0.347784488239777,
-0.7358));
#65956=CARTESIAN_POINT('Ctrl Pts',(0.262319512338524,-0.35058249836084,
-0.7358));
#65957=CARTESIAN_POINT('Ctrl Pts',(0.258103949731175,-0.353310108913971,
-0.7358));
#65958=CARTESIAN_POINT('Ctrl Pts',(0.253835875722689,-0.355965150255044,
-0.7358));
#65959=CARTESIAN_POINT('Ctrl Pts',(0.287047174344898,-0.402732536982762,
-0.768920421448668));
#65960=CARTESIAN_POINT('Ctrl Pts',(0.353806905076701,-0.355150314361416,
-0.766282186574675));
#65961=CARTESIAN_POINT('Ctrl Pts',(0.462114121615473,-0.226365817495061,
-0.761006923386275));
#65962=CARTESIAN_POINT('Ctrl Pts',(0.534659959470215,0.105244592708357,
-0.750457603569065));
#65963=CARTESIAN_POINT('Ctrl Pts',(0.297699882545806,0.502243459957053,
-0.737272461997036));
#65964=CARTESIAN_POINT('Ctrl Pts',(-0.259650455921768,0.523296542714125,
-0.721450292110602));
#65965=CARTESIAN_POINT('Ctrl Pts',(-0.579765127206865,0.0677026564476974,
-0.705628122224166));
#65966=CARTESIAN_POINT('Ctrl Pts',(-0.37310450485665,-0.449122313750527,
-0.689805952337734));
#65967=CARTESIAN_POINT('Ctrl Pts',(0.173195203905992,-0.55762972329304,
-0.673983782451298));
#65968=CARTESIAN_POINT('Ctrl Pts',(0.561818783331492,-0.158854163257542,
-0.658161612564864));
#65969=CARTESIAN_POINT('Ctrl Pts',(0.439518970328374,0.38435807019179,-0.642339442678429));
#65970=CARTESIAN_POINT('Ctrl Pts',(-0.0825831408533865,0.578004249452697,
-0.626517272791996));
#65971=CARTESIAN_POINT('Ctrl Pts',(-0.529551478372892,0.245916087209467,
-0.61069510290556));
#65972=CARTESIAN_POINT('Ctrl Pts',(-0.494879278247576,-0.309837196314249,
-0.594872933019126));
#65973=CARTESIAN_POINT('Ctrl Pts',(-0.010086200220884,-0.583782926351103,
-0.579050763132692));
#65974=CARTESIAN_POINT('Ctrl Pts',(0.483877844048874,-0.326749585733395,
-0.563228593246258));
#65975=CARTESIAN_POINT('Ctrl Pts',(0.537734390222952,0.227476475521788,
-0.547406423359823));
#65976=CARTESIAN_POINT('Ctrl Pts',(0.102496165195714,0.57480278682962,-0.531584253473389));
#65977=CARTESIAN_POINT('Ctrl Pts',(-0.425966598017122,0.399319450617198,
-0.515762083586955));
#65978=CARTESIAN_POINT('Ctrl Pts',(-0.566993494230472,-0.139363031519207,
-0.499939913700521));
#65979=CARTESIAN_POINT('Ctrl Pts',(-0.192313798984891,-0.551288541463694,
-0.484117743814086));
#65980=CARTESIAN_POINT('Ctrl Pts',(0.357284023531408,-0.461791902996352,
-0.468295573927652));
#65981=CARTESIAN_POINT('Ctrl Pts',(0.581915737174481,0.0477255410775767,
-0.452473404041217));
#65982=CARTESIAN_POINT('Ctrl Pts',(0.27726849072569,0.513834444634811,-0.436651234154783));
#65983=CARTESIAN_POINT('Ctrl Pts',(-0.27956710218963,0.512587427193721,
-0.420829064268349));
#65984=CARTESIAN_POINT('Ctrl Pts',(-0.58212365522641,0.0451187683232971,
-0.405006894381914));
#65985=CARTESIAN_POINT('Ctrl Pts',(-0.355212141653185,-0.463387539189459,
-0.38918472449548));
#65986=CARTESIAN_POINT('Ctrl Pts',(0.194781019166425,-0.550421584642162,
-0.373362554609046));
#65987=CARTESIAN_POINT('Ctrl Pts',(0.567611984296084,-0.136822304140763,
-0.357540384722611));
#65988=CARTESIAN_POINT('Ctrl Pts',(0.42417384978651,0.401223586671516,-0.341718214836177));
#65989=CARTESIAN_POINT('Ctrl Pts',(-0.10506963626688,0.574337384533757,
-0.325896044949742));
#65990=CARTESIAN_POINT('Ctrl Pts',(-0.538747758010019,0.225066856229725,
-0.310073875063308));
#65991=CARTESIAN_POINT('Ctrl Pts',(-0.482409667299879,-0.328915644435373,
-0.294251705176874));
#65992=CARTESIAN_POINT('Ctrl Pts',(0.012701054010981,-0.583727824779955,
-0.278429535290439));
#65993=CARTESIAN_POINT('Ctrl Pts',(0.496261505533139,-0.30762543078323,
-0.262607365404005));
#65994=CARTESIAN_POINT('Ctrl Pts',(0.528445756192563,0.248300491667137,
-0.246785195517571));
#65995=CARTESIAN_POINT('Ctrl Pts',(0.079991563384182,0.578339295116359,
-0.230963025631136));
#65996=CARTESIAN_POINT('Ctrl Pts',(-0.441232296079768,0.382441561355567,
-0.215140855744702));
#65997=CARTESIAN_POINT('Ctrl Pts',(-0.561108876051582,-0.161476479615712,
-0.199318685858268));
#65998=CARTESIAN_POINT('Ctrl Pts',(-0.170682109742751,-0.558192502483715,
-0.183496515971833));
#65999=CARTESIAN_POINT('Ctrl Pts',(0.375086411458179,-0.447847981815665,
-0.167674346085399));
#66000=CARTESIAN_POINT('Ctrl Pts',(0.57949957025952,0.071091217505752,-0.151852176198965));
#66001=CARTESIAN_POINT('Ctrl Pts',(0.310985042693996,0.44746619959015,-0.138667034626936));
#66002=CARTESIAN_POINT('Ctrl Pts',(-0.0218228806034698,0.514106220352834,
-0.128118921369313));
#66003=CARTESIAN_POINT('Ctrl Pts',(-0.183213450909262,0.466623101184697,
-0.122844864740502));
#66004=CARTESIAN_POINT('Ctrl Pts',(-0.253566780180828,0.424609779704417,
-0.120207836426096));
#66005=CARTESIAN_POINT('Ctrl Pts',(0.275865587548243,-0.387044562250431,
-0.757797765364769));
#66006=CARTESIAN_POINT('Ctrl Pts',(0.340024771086357,-0.341315849434336,
-0.755159530490776));
#66007=CARTESIAN_POINT('Ctrl Pts',(0.444113006737419,-0.217548001949956,
-0.749884267302376));
#66008=CARTESIAN_POINT('Ctrl Pts',(0.513832906365942,0.101144912748319,
-0.739334947485166));
#66009=CARTESIAN_POINT('Ctrl Pts',(0.286103331966143,0.482679153660087,
-0.726149805913137));
#66010=CARTESIAN_POINT('Ctrl Pts',(-0.249536076233809,0.502912138213013,
-0.710327636026703));
#66011=CARTESIAN_POINT('Ctrl Pts',(-0.557181055071921,0.0650653786860826,
-0.694505466140268));
#66012=CARTESIAN_POINT('Ctrl Pts',(-0.358570655447406,-0.431627279545863,
-0.678683296253835));
#66013=CARTESIAN_POINT('Ctrl Pts',(0.166448587397194,-0.535907909916455,
-0.662861126367399));
#66014=CARTESIAN_POINT('Ctrl Pts',(0.539933790022817,-0.152666185206451,
-0.647038956480965));
#66015=CARTESIAN_POINT('Ctrl Pts',(0.422398023129646,0.36938585131295,-0.631216786594532));
#66016=CARTESIAN_POINT('Ctrl Pts',(-0.0793662112337171,0.555488770250224,
-0.615394616708097));
#66017=CARTESIAN_POINT('Ctrl Pts',(-0.508923420172224,0.236336713783819,
-0.599572446821662));
#66018=CARTESIAN_POINT('Ctrl Pts',(-0.475601835032119,-0.297767850878864,
-0.583750276935229));
#66019=CARTESIAN_POINT('Ctrl Pts',(-0.00969330409335463,-0.561042345551805,
-0.567928107048793));
#66020=CARTESIAN_POINT('Ctrl Pts',(0.465028948829617,-0.31402143795773,
-0.55210593716236));
#66021=CARTESIAN_POINT('Ctrl Pts',(0.516787576266163,0.218615395592856,
-0.536283767275924));
#66022=CARTESIAN_POINT('Ctrl Pts',(0.0985035470134388,0.552412016857531,
-0.520461597389491));
#66023=CARTESIAN_POINT('Ctrl Pts',(-0.409373567623862,0.383764428670513,
-0.504639427503056));
#66024=CARTESIAN_POINT('Ctrl Pts',(-0.544906926113765,-0.133934307697998,
-0.488817257616623));
#66025=CARTESIAN_POINT('Ctrl Pts',(-0.184822439975864,-0.529813741405321,
-0.472995087730187));
#66026=CARTESIAN_POINT('Ctrl Pts',(0.343366442460311,-0.44380333976757,
-0.457172917843752));
#66027=CARTESIAN_POINT('Ctrl Pts',(0.559247890544722,0.0458664484695617,
-0.44135074795732));
#66028=CARTESIAN_POINT('Ctrl Pts',(0.266467821107177,0.493818625092579,
-0.425528578070885));
#66029=CARTESIAN_POINT('Ctrl Pts',(-0.268676892851193,0.492620183756744,
-0.409706408184451));
#66030=CARTESIAN_POINT('Ctrl Pts',(-0.559447709392226,0.0433612194976846,
-0.393884238298015));
#66031=CARTESIAN_POINT('Ctrl Pts',(-0.341375268316301,-0.445336819819863,
-0.378062068411582));
#66032=CARTESIAN_POINT('Ctrl Pts',(0.187193552482174,-0.528980555872327,
-0.362239898525148));
#66033=CARTESIAN_POINT('Ctrl Pts',(0.545501323622579,-0.131492551381623,
-0.346417728638712));
#66034=CARTESIAN_POINT('Ctrl Pts',(0.407650653802841,0.385594391332905,
-0.330595558752279));
#66035=CARTESIAN_POINT('Ctrl Pts',(-0.100976771530301,0.551964743763527,
-0.314773388865843));
#66036=CARTESIAN_POINT('Ctrl Pts',(-0.517761469496849,0.21629964020077,
-0.29895121897941));
#66037=CARTESIAN_POINT('Ctrl Pts',(-0.463617963187935,-0.316103120377524,
-0.283129049092976));
#66038=CARTESIAN_POINT('Ctrl Pts',(0.0122062993137546,-0.560989390397886,
-0.26730687920654));
#66039=CARTESIAN_POINT('Ctrl Pts',(0.476930219271146,-0.295642242086072,
-0.251484709320108));
#66040=CARTESIAN_POINT('Ctrl Pts',(0.507860770105602,0.238628236555884,
-0.235662539433672));
#66041=CARTESIAN_POINT('Ctrl Pts',(0.0768755856323659,0.555810764602103,
-0.219840369547239));
#66042=CARTESIAN_POINT('Ctrl Pts',(-0.424044608281193,0.367543997835894,
-0.204018199660804));
#66043=CARTESIAN_POINT('Ctrl Pts',(-0.539251536350318,-0.155186352299316,
-0.18819602977437));
#66044=CARTESIAN_POINT('Ctrl Pts',(-0.164033387876457,-0.536448766702277,
-0.172373859887935));
#66045=CARTESIAN_POINT('Ctrl Pts',(0.360475359196343,-0.4304025877204,-0.156551690001501));
#66046=CARTESIAN_POINT('Ctrl Pts',(0.556925842584725,0.068321942313148,
-0.140729520115067));
#66047=CARTESIAN_POINT('Ctrl Pts',(0.298870984246006,0.43003567737475,-0.127544378543038));
#66048=CARTESIAN_POINT('Ctrl Pts',(-0.0209727958249744,0.494079814105516,
-0.116996265285415));
#66049=CARTESIAN_POINT('Ctrl Pts',(-0.176076585311013,0.448446344283576,
-0.111722208656604));
#66050=CARTESIAN_POINT('Ctrl Pts',(-0.243689382962719,0.408069602580887,
-0.109085180342198));
#66051=CARTESIAN_POINT('Ctrl Pts',(0.264684000751588,-0.371356587518099,
-0.746675109280871));
#66052=CARTESIAN_POINT('Ctrl Pts',(0.326242637096013,-0.327481384507258,
-0.744036874406877));
#66053=CARTESIAN_POINT('Ctrl Pts',(0.426111891859364,-0.208730186404851,
-0.738761611218477));
#66054=CARTESIAN_POINT('Ctrl Pts',(0.493005853261671,0.0970452327882826,
-0.728212291401267));
#66055=CARTESIAN_POINT('Ctrl Pts',(0.274506781386479,0.463114847363122,
-0.715027149829239));
#66056=CARTESIAN_POINT('Ctrl Pts',(-0.239421696545848,0.482527733711901,
-0.699204979942805));
#66057=CARTESIAN_POINT('Ctrl Pts',(-0.534596982936976,0.0624281009244681,
-0.68338281005637));
#66058=CARTESIAN_POINT('Ctrl Pts',(-0.344036806038162,-0.414132245341199,
-0.667560640169936));
#66059=CARTESIAN_POINT('Ctrl Pts',(0.159701970888396,-0.51418609653987,
-0.651738470283501));
#66060=CARTESIAN_POINT('Ctrl Pts',(0.518048796714141,-0.146478207155357,
-0.635916300397068));
#66061=CARTESIAN_POINT('Ctrl Pts',(0.405277075930918,0.35441363243411,-0.620094130510632));
#66062=CARTESIAN_POINT('Ctrl Pts',(-0.0761492816140481,0.532973291047753,
-0.604271960624199));
#66063=CARTESIAN_POINT('Ctrl Pts',(-0.488295361971557,0.226757340358172,
-0.588449790737764));
#66064=CARTESIAN_POINT('Ctrl Pts',(-0.456324391816661,-0.285698505443478,
-0.57262762085133));
#66065=CARTESIAN_POINT('Ctrl Pts',(-0.00930040796582533,-0.538301764752508,
-0.556805450964895));
#66066=CARTESIAN_POINT('Ctrl Pts',(0.44618005361036,-0.301293290182064,
-0.540983281078462));
#66067=CARTESIAN_POINT('Ctrl Pts',(0.495840762309375,0.209754315663926,
-0.525161111192026));
#66068=CARTESIAN_POINT('Ctrl Pts',(0.0945109288311632,0.530021246885443,
-0.509338941305593));
#66069=CARTESIAN_POINT('Ctrl Pts',(-0.392780537230601,0.368209406723828,
-0.493516771419158));
#66070=CARTESIAN_POINT('Ctrl Pts',(-0.522820357997059,-0.128505583876788,
-0.477694601532724));
#66071=CARTESIAN_POINT('Ctrl Pts',(-0.177331080966838,-0.508338941346947,
-0.461872431646289));
#66072=CARTESIAN_POINT('Ctrl Pts',(0.329448861389214,-0.425814776538789,
-0.446050261759855));
#66073=CARTESIAN_POINT('Ctrl Pts',(0.536580043914961,0.0440073558615464,
-0.430228091873421));
#66074=CARTESIAN_POINT('Ctrl Pts',(0.255667151488665,0.473802805550347,
-0.414405921986986));
#66075=CARTESIAN_POINT('Ctrl Pts',(-0.257786683512757,0.472652940319767,
-0.398583752100552));
#66076=CARTESIAN_POINT('Ctrl Pts',(-0.536771763558043,0.0416036706720726,
-0.382761582214118));
#66077=CARTESIAN_POINT('Ctrl Pts',(-0.327538394979417,-0.427286100450265,
-0.366939412327683));
#66078=CARTESIAN_POINT('Ctrl Pts',(0.179606085797923,-0.507539527102493,
-0.351117242441249));
#66079=CARTESIAN_POINT('Ctrl Pts',(0.523390662949075,-0.126162798622482,
-0.335295072554814));
#66080=CARTESIAN_POINT('Ctrl Pts',(0.391127457819172,0.369965195994294,
-0.31947290266838));
#66081=CARTESIAN_POINT('Ctrl Pts',(-0.0968839067937205,0.529592102993296,
-0.303650732781946));
#66082=CARTESIAN_POINT('Ctrl Pts',(-0.496775180983678,0.207532424171815,
-0.287828562895511));
#66083=CARTESIAN_POINT('Ctrl Pts',(-0.444826259075989,-0.303290596319674,
-0.272006393009077));
#66084=CARTESIAN_POINT('Ctrl Pts',(0.0117115446165282,-0.538250956015816,
-0.256184223122643));
#66085=CARTESIAN_POINT('Ctrl Pts',(0.457598933009152,-0.283659053388913,
-0.240362053236208));
#66086=CARTESIAN_POINT('Ctrl Pts',(0.487275784018641,0.228955981444631,
-0.224539883349774));
#66087=CARTESIAN_POINT('Ctrl Pts',(0.0737596078805499,0.533282234087846,
-0.20871771346334));
#66088=CARTESIAN_POINT('Ctrl Pts',(-0.406856920482618,0.352646434316222,
-0.192895543576905));
#66089=CARTESIAN_POINT('Ctrl Pts',(-0.517394196649054,-0.148896224982918,
-0.177073373690471));
#66090=CARTESIAN_POINT('Ctrl Pts',(-0.157384666010164,-0.514705030920839,
-0.161251203804036));
#66091=CARTESIAN_POINT('Ctrl Pts',(0.345864306934509,-0.412957193625136,
-0.145429033917602));
#66092=CARTESIAN_POINT('Ctrl Pts',(0.534352114909929,0.0655526671205438,
-0.129606864031168));
#66093=CARTESIAN_POINT('Ctrl Pts',(0.286756925798016,0.412605155159349,
-0.116421722459139));
#66094=CARTESIAN_POINT('Ctrl Pts',(-0.0201227110464791,0.474053407858199,
-0.105873609201516));
#66095=CARTESIAN_POINT('Ctrl Pts',(-0.168939719712765,0.430269587382454,
-0.100599552572705));
#66096=CARTESIAN_POINT('Ctrl Pts',(-0.23381198574461,0.391529425457356,
-0.0979625242582989));
#66097=CARTESIAN_POINT('Ctrl Pts',(0.253502413954933,-0.355668612785768,
-0.735552453196972));
#66098=CARTESIAN_POINT('Ctrl Pts',(0.312460503105669,-0.313646919580179,
-0.732914218322978));
#66099=CARTESIAN_POINT('Ctrl Pts',(0.40811077698131,-0.199912370859746,
-0.727638955134579));
#66100=CARTESIAN_POINT('Ctrl Pts',(0.4721788001574,0.0929455528282454,-0.717089635317369));
#66101=CARTESIAN_POINT('Ctrl Pts',(0.262910230806816,0.443550541066156,
-0.70390449374534));
#66102=CARTESIAN_POINT('Ctrl Pts',(-0.229307316857889,0.462143329210789,
-0.688082323858905));
#66103=CARTESIAN_POINT('Ctrl Pts',(-0.512012910802029,0.0597908231628538,
-0.672260153972472));
#66104=CARTESIAN_POINT('Ctrl Pts',(-0.329502956628918,-0.396637211136535,
-0.656437984086036));
#66105=CARTESIAN_POINT('Ctrl Pts',(0.152955354379598,-0.492464283163283,
-0.640615814199603));
#66106=CARTESIAN_POINT('Ctrl Pts',(0.496163803405466,-0.140290229104266,
-0.624793644313168));
#66107=CARTESIAN_POINT('Ctrl Pts',(0.388156128732189,0.339441413555271,
-0.608971474426735));
#66108=CARTESIAN_POINT('Ctrl Pts',(-0.0729323519943785,0.510457811845281,
-0.593149304540299));
#66109=CARTESIAN_POINT('Ctrl Pts',(-0.467667303770891,0.217177966932526,
-0.577327134653866));
#66110=CARTESIAN_POINT('Ctrl Pts',(-0.437046948601204,-0.273629160008092,
-0.56150496476743));
#66111=CARTESIAN_POINT('Ctrl Pts',(-0.00890751183829607,-0.51556118395321,
-0.545682794880997));
#66112=CARTESIAN_POINT('Ctrl Pts',(0.427331158391103,-0.288565142406399,
-0.529860624994562));
#66113=CARTESIAN_POINT('Ctrl Pts',(0.474893948352587,0.200893235734995,
-0.514038455108128));
#66114=CARTESIAN_POINT('Ctrl Pts',(0.0905183106488877,0.507630476913353,
-0.498216285221693));
#66115=CARTESIAN_POINT('Ctrl Pts',(-0.376187506837341,0.352654384777143,
-0.482394115335259));
#66116=CARTESIAN_POINT('Ctrl Pts',(-0.500733789880351,-0.12307686005558,
-0.466571945448824));
#66117=CARTESIAN_POINT('Ctrl Pts',(-0.169839721957813,-0.486864141288574,
-0.450749775562391));
#66118=CARTESIAN_POINT('Ctrl Pts',(0.315531280318115,-0.407826213310007,
-0.434927605675956));
#66119=CARTESIAN_POINT('Ctrl Pts',(0.513912197285202,0.0421482632535317,
-0.419105435789522));
#66120=CARTESIAN_POINT('Ctrl Pts',(0.244866481870151,0.453786986008114,
-0.403283265903088));
#66121=CARTESIAN_POINT('Ctrl Pts',(-0.24689647417432,0.452685696882792,
-0.387461096016653));
#66122=CARTESIAN_POINT('Ctrl Pts',(-0.514095817723861,0.0398461218464604,
-0.371638926130219));
#66123=CARTESIAN_POINT('Ctrl Pts',(-0.313701521642532,-0.409235381080669,
-0.355816756243784));
#66124=CARTESIAN_POINT('Ctrl Pts',(0.172018619113672,-0.486098498332657,
-0.33999458635735));
#66125=CARTESIAN_POINT('Ctrl Pts',(0.501280002275571,-0.12083304586334,
-0.324172416470915));
#66126=CARTESIAN_POINT('Ctrl Pts',(0.374604261835502,0.354336000655682,
-0.308350246584481));
#66127=CARTESIAN_POINT('Ctrl Pts',(-0.0927910420571407,0.507219462223066,
-0.292528076698047));
#66128=CARTESIAN_POINT('Ctrl Pts',(-0.475788892470508,0.198765208142859,
-0.276705906811612));
#66129=CARTESIAN_POINT('Ctrl Pts',(-0.426034554964045,-0.290478072261824,
-0.260883736925178));
#66130=CARTESIAN_POINT('Ctrl Pts',(0.0112167899193015,-0.515512521633748,
-0.245061567038744));
#66131=CARTESIAN_POINT('Ctrl Pts',(0.438267646747159,-0.271675864691754,
-0.229239397152309));
#66132=CARTESIAN_POINT('Ctrl Pts',(0.46669079793168,0.219283726333378,-0.213417227265875));
#66133=CARTESIAN_POINT('Ctrl Pts',(0.0706436301287334,0.510753703573591,
-0.197595057379441));
#66134=CARTESIAN_POINT('Ctrl Pts',(-0.389669232684042,0.33774887079655,
-0.181772887493006));
#66135=CARTESIAN_POINT('Ctrl Pts',(-0.495536856947789,-0.142606097666521,
-0.165950717606572));
#66136=CARTESIAN_POINT('Ctrl Pts',(-0.150735944143869,-0.492961295139401,
-0.150128547720138));
#66137=CARTESIAN_POINT('Ctrl Pts',(0.331253254672673,-0.395511799529872,
-0.134306377833703));
#66138=CARTESIAN_POINT('Ctrl Pts',(0.511778387235135,0.0627833919279398,
-0.118484207947269));
#66139=CARTESIAN_POINT('Ctrl Pts',(0.274642867350025,0.395174632943949,
-0.10529906637524));
#66140=CARTESIAN_POINT('Ctrl Pts',(-0.0192726262679835,0.454027001610881,
-0.0947509531176172));
#66141=CARTESIAN_POINT('Ctrl Pts',(-0.161802854114516,0.412092830481332,
-0.0894768964888058));
#66142=CARTESIAN_POINT('Ctrl Pts',(-0.223934588526501,0.374989248333826,
-0.0868398681744001));
#66143=CARTESIAN_POINT('',(0.435851714755768,0.0627985268057629,-0.120000000000001));
#66144=CARTESIAN_POINT('Ctrl Pts',(0.436962529762211,0.0516115063121503,
-0.12));
#66145=CARTESIAN_POINT('Ctrl Pts',(0.436592258093396,0.0553405131433545,
-0.12));
#66146=CARTESIAN_POINT('Ctrl Pts',(0.436221986424582,0.0590695199745587,
-0.12));
#66147=CARTESIAN_POINT('Ctrl Pts',(0.435851714755768,0.0627985268057629,
-0.12));
#66148=CARTESIAN_POINT('Ctrl Pts',(0.228820166259496,0.438035354181574,
-0.7358));
#66149=CARTESIAN_POINT('Ctrl Pts',(0.22491465564395,0.440009924652994,-0.7358));
#66150=CARTESIAN_POINT('Ctrl Pts',(0.221009145028404,0.441984495124415,
-0.7358));
#66151=CARTESIAN_POINT('Ctrl Pts',(0.217103634412858,0.443959065595836,
-0.7358));
#66152=CARTESIAN_POINT('Ctrl Pts',(0.436199126192416,0.0628594907761131,
-0.120000000000003));
#66153=CARTESIAN_POINT('Ctrl Pts',(0.434282017858336,0.0862483264787582,
-0.120000000000003));
#66154=CARTESIAN_POINT('Ctrl Pts',(0.430334856380413,0.109415622186605,
-0.120000000000002));
#66155=CARTESIAN_POINT('Ctrl Pts',(0.424527759942032,0.132185099075521,
-0.120000000000001));
#66156=CARTESIAN_POINT('Ctrl Pts',(0.420100481655662,0.149544344214974,
-0.120000000000001));
#66157=CARTESIAN_POINT('Ctrl Pts',(0.414590868119256,0.166672689290124,
-0.120000000000001));
#66158=CARTESIAN_POINT('Ctrl Pts',(0.408054534382917,0.18348953378457,-0.120000000000001));
#66159=CARTESIAN_POINT('Ctrl Pts',(0.40502540392714,0.191282957113767,-0.120000000000001));
#66160=CARTESIAN_POINT('Ctrl Pts',(0.401780759259403,0.198995404037311,
-0.12));
#66161=CARTESIAN_POINT('Ctrl Pts',(0.398332969755228,0.206608400908161,
-0.12));
#66162=CARTESIAN_POINT('Ctrl Pts',(0.388174784716126,0.229038491498828,
-0.120000000000001));
#66163=CARTESIAN_POINT('Ctrl Pts',(0.376245486250458,0.250636268527475,
-0.120000000000001));
#66164=CARTESIAN_POINT('Ctrl Pts',(0.362715113103607,0.271207164179327,
-0.120000000000001));
#66165=CARTESIAN_POINT('Ctrl Pts',(0.352729984400094,0.286388049318335,
-0.12));
#66166=CARTESIAN_POINT('Ctrl Pts',(0.341871626615223,0.301009751788514,
-0.12));
#66167=CARTESIAN_POINT('Ctrl Pts',(0.33019145063168,0.31498725114189,-0.12));
#66168=CARTESIAN_POINT('Ctrl Pts',(0.325584301106223,0.320500561010141,
-0.120000000000001));
#66169=CARTESIAN_POINT('Ctrl Pts',(0.320849147972658,0.325913550689098,
-0.120000000000001));
#66170=CARTESIAN_POINT('Ctrl Pts',(0.315988625581974,0.331220579977179,
-0.120000000000001));
#66171=CARTESIAN_POINT('Ctrl Pts',(0.311350868263747,0.336284380108213,
-0.120000000000001));
#66172=CARTESIAN_POINT('Ctrl Pts',(0.306602392532854,0.34124766516251,-0.120000000000001));
#66173=CARTESIAN_POINT('Ctrl Pts',(0.30175612487152,0.346096268998127,-0.120000000000001));
#66174=CARTESIAN_POINT('Ctrl Pts',(0.291874915505376,0.355982241664367,
-0.12));
#66175=CARTESIAN_POINT('Ctrl Pts',(0.281576313869693,0.365403929425632,
-0.12));
#66176=CARTESIAN_POINT('Ctrl Pts',(0.270887565775841,0.374326851892634,
-0.12));
#66177=CARTESIAN_POINT('Ctrl Pts',(0.251903626591773,0.390174565391949,
-0.12));
#66178=CARTESIAN_POINT('Ctrl Pts',(0.231691070691565,0.40445115675579,-0.12));
#66179=CARTESIAN_POINT('Ctrl Pts',(0.210372408766704,0.416938641833649,
-0.120000000000001));
#66180=CARTESIAN_POINT('Ctrl Pts',(0.208825510914833,0.417844742972186,
-0.120000000000001));
#66181=CARTESIAN_POINT('Ctrl Pts',(0.207272774284322,0.418741407052641,
-0.12));
#66182=CARTESIAN_POINT('Ctrl Pts',(0.205714238886768,0.419628542173557,
-0.12));
#66183=CARTESIAN_POINT('Ctrl Pts',(0.194936314682677,0.425763452620268,
-0.12));
#66184=CARTESIAN_POINT('Ctrl Pts',(0.183881198468354,0.431442908347822,
-0.12));
#66185=CARTESIAN_POINT('Ctrl Pts',(0.172580759002838,0.436664729050456,
-0.12));
#66186=CARTESIAN_POINT('Ctrl Pts',(0.166054055780333,0.439680653706417,
-0.12));
#66187=CARTESIAN_POINT('Ctrl Pts',(0.159448793534031,0.442542034058426,
-0.12));
#66188=CARTESIAN_POINT('Ctrl Pts',(0.152787789335078,0.445242616657749,
-0.12));
#66189=CARTESIAN_POINT('Ctrl Pts',(0.129789624052855,0.454566803090074,
-0.12));
#66190=CARTESIAN_POINT('Ctrl Pts',(0.106076488766298,0.462002433444808,
-0.12));
#66191=CARTESIAN_POINT('Ctrl Pts',(0.0819188252479975,0.467568632172314,
-0.12));
#66192=CARTESIAN_POINT('Ctrl Pts',(0.0652486944624254,0.471409618726982,
-0.12));
#66193=CARTESIAN_POINT('Ctrl Pts',(0.0483660449802322,0.474359558588752,
-0.12));
#66194=CARTESIAN_POINT('Ctrl Pts',(0.0313536819883358,0.476412263640607,
-0.12));
#66195=CARTESIAN_POINT('Ctrl Pts',(0.0210620943032514,0.477654042577657,
-0.12));
#66196=CARTESIAN_POINT('Ctrl Pts',(0.0107229630418266,0.478567267564897,
-0.119999999999999));
#66197=CARTESIAN_POINT('Ctrl Pts',(0.000354321129172847,0.479148654832135,
-0.12));
#66198=CARTESIAN_POINT('Ctrl Pts',(-0.00641677334760411,0.479528321537498,
-0.12));
#66199=CARTESIAN_POINT('Ctrl Pts',(-0.0132040195152825,0.479766395875062,
-0.12));
#66200=CARTESIAN_POINT('Ctrl Pts',(-0.0199846559383493,0.479861665078788,
-0.12));
#66201=CARTESIAN_POINT('Ctrl Pts',(-0.0402355271055921,0.48014619358769,
-0.12));
#66202=CARTESIAN_POINT('Ctrl Pts',(-0.0604463821016128,0.479160928462546,
-0.12));
#66203=CARTESIAN_POINT('Ctrl Pts',(-0.0805127730529895,0.476939899349321,
-0.12));
#66204=CARTESIAN_POINT('Ctrl Pts',(-0.0927943658103894,0.475580523109864,
-0.119999999999999));
#66205=CARTESIAN_POINT('Ctrl Pts',(-0.105021940048514,0.473757828575607,
-0.12));
#66206=CARTESIAN_POINT('Ctrl Pts',(-0.117171754670614,0.471475909875768,
-0.12));
#66207=CARTESIAN_POINT('Ctrl Pts',(-0.129239401322921,0.469209423561742,
-0.12));
#66208=CARTESIAN_POINT('Ctrl Pts',(-0.141237375343505,0.466487419270226,
-0.12));
#66209=CARTESIAN_POINT('Ctrl Pts',(-0.153098179736105,0.463324713469219,
-0.12));
#66210=CARTESIAN_POINT('Ctrl Pts',(-0.178118993169746,0.456652866503944,
-0.12));
#66211=CARTESIAN_POINT('Ctrl Pts',(-0.202564229149912,0.448019164461463,
-0.12));
#66212=CARTESIAN_POINT('Ctrl Pts',(-0.226217519016056,0.437461691518522,
-0.12));
#66213=CARTESIAN_POINT('Ctrl Pts',(-0.235396166019609,0.433364869556706,
-0.12));
#66214=CARTESIAN_POINT('Ctrl Pts',(-0.244455472878046,0.428977817680041,
-0.12));
#66215=CARTESIAN_POINT('Ctrl Pts',(-0.253382212491109,0.424300712223195,
-0.12));
#66216=CARTESIAN_POINT('Origin',(0.,0.,0.3066185719505));
#66217=CARTESIAN_POINT('',(-0.25,0.144337567297406,0.288452994616207));
#66218=CARTESIAN_POINT('',(-0.25,-3.42699144208774E-17,0.266123895246948));
#66219=CARTESIAN_POINT('Ctrl Pts',(-0.25,0.144337567297406,0.288452994616208));
#66220=CARTESIAN_POINT('Ctrl Pts',(-0.25,0.0669872981077807,0.266123895246948));
#66221=CARTESIAN_POINT('Ctrl Pts',(-0.25,-3.79236588630711E-17,0.266123895246948));
#66222=CARTESIAN_POINT('',(1.76762539787485E-17,0.288675134594813,0.288452994616207));
#66223=CARTESIAN_POINT('Ctrl Pts',(1.76762539787485E-17,0.288675134594813,
0.288452994616207));
#66224=CARTESIAN_POINT('Ctrl Pts',(-0.125,0.21650635094611,0.246786327949541));
#66225=CARTESIAN_POINT('Ctrl Pts',(-0.25,0.144337567297406,0.288452994616207));
#66226=CARTESIAN_POINT('',(0.25,0.144337567297406,0.288452994616207));
#66227=CARTESIAN_POINT('Ctrl Pts',(0.25,0.144337567297406,0.288452994616207));
#66228=CARTESIAN_POINT('Ctrl Pts',(0.125,0.21650635094611,0.246786327949541));
#66229=CARTESIAN_POINT('Ctrl Pts',(1.76762539787484E-17,0.288675134594813,
0.288452994616207));
#66230=CARTESIAN_POINT('',(0.25,-0.144337567297407,0.288452994616207));
#66231=CARTESIAN_POINT('Ctrl Pts',(0.25,-0.144337567297407,0.288452994616207));
#66232=CARTESIAN_POINT('Ctrl Pts',(0.25,1.66533453693773E-16,0.246786327949541));
#66233=CARTESIAN_POINT('Ctrl Pts',(0.25,0.144337567297406,0.288452994616207));
#66234=CARTESIAN_POINT('',(-5.30287619362453E-17,-0.288675134594813,0.288452994616207));
#66235=CARTESIAN_POINT('Ctrl Pts',(-5.30287619362453E-17,-0.288675134594813,
0.288452994616207));
#66236=CARTESIAN_POINT('Ctrl Pts',(0.125,-0.21650635094611,0.246786327949541));
#66237=CARTESIAN_POINT('Ctrl Pts',(0.25,-0.144337567297407,0.288452994616207));
#66238=CARTESIAN_POINT('',(-0.25,-0.144337567297406,0.288452994616207));
#66239=CARTESIAN_POINT('Ctrl Pts',(-0.25,-0.144337567297406,0.288452994616207));
#66240=CARTESIAN_POINT('Ctrl Pts',(-0.125,-0.21650635094611,0.246786327949541));
#66241=CARTESIAN_POINT('Ctrl Pts',(-5.30287619362453E-17,-0.288675134594813,
0.288452994616207));
#66242=CARTESIAN_POINT('Ctrl Pts',(-0.25,-3.79236588630711E-17,0.266123895246948));
#66243=CARTESIAN_POINT('Ctrl Pts',(-0.25,-0.0669872981077806,0.266123895246948));
#66244=CARTESIAN_POINT('Ctrl Pts',(-0.25,-0.144337567297406,0.288452994616208));
#66245=CARTESIAN_POINT('',(-0.308675134594813,3.78018015557916E-17,0.3));
#66246=CARTESIAN_POINT('',(-0.320138837486628,-3.92057002610754E-17,0.3066185719505));
#66247=CARTESIAN_POINT('Origin',(0.,0.,0.3));
#66248=CARTESIAN_POINT('Origin',(-5.55111512312578E-17,-0.288675134594813,
0.3));
#66249=CARTESIAN_POINT('',(-5.55111512312578E-17,-0.288675134594813,-5.55111512312578E-17));
#66250=CARTESIAN_POINT('',(-5.30287619362453E-17,-0.288675134594813,0.3));
#66251=CARTESIAN_POINT('',(-0.25,-0.144337567297406,-5.55111512312578E-17));
#66252=CARTESIAN_POINT('',(-0.25,-0.144337567297406,-5.55111512312578E-17));
#66253=CARTESIAN_POINT('',(-0.25,-0.144337567297406,0.3));
#66254=CARTESIAN_POINT('Origin',(0.25,-0.144337567297407,0.3));
#66255=CARTESIAN_POINT('',(0.25,-0.144337567297407,-5.55111512312578E-17));
#66256=CARTESIAN_POINT('',(0.25,-0.144337567297407,0.3));
#66257=CARTESIAN_POINT('',(-5.30287619362453E-17,-0.288675134594813,-5.55111512312578E-17));
#66258=CARTESIAN_POINT('Origin',(0.25,0.144337567297406,0.3));
#66259=CARTESIAN_POINT('',(0.25,0.144337567297406,-5.55111512312578E-17));
#66260=CARTESIAN_POINT('',(0.25,0.144337567297406,0.3));
#66261=CARTESIAN_POINT('',(0.25,-0.144337567297407,-5.55111512312578E-17));
#66262=CARTESIAN_POINT('Origin',(0.,0.,-0.0731054258308761));
#66263=CARTESIAN_POINT('',(0.,0.,-0.147210851661752));
#66264=CARTESIAN_POINT('',(-0.243346949651439,2.98014062972907E-17,-5.55111512312578E-17));
#66265=CARTESIAN_POINT('',(-0.1225,-1.50019232895551E-17,-0.0731054258308761));
#66266=CARTESIAN_POINT('Origin',(0.,0.,-5.55111512312578E-17));
#66267=CARTESIAN_POINT('Origin',(0.,0.288675134594813,0.3));
#66268=CARTESIAN_POINT('',(2.77555756156289E-17,0.288675134594813,-5.55111512312578E-17));
#66269=CARTESIAN_POINT('',(1.76762539787485E-17,0.288675134594813,0.3));
#66270=CARTESIAN_POINT('',(0.25,0.144337567297406,-5.55111512312578E-17));
#66271=CARTESIAN_POINT('Origin',(-0.25,0.144337567297406,0.3));
#66272=CARTESIAN_POINT('',(-0.25,0.144337567297406,-5.55111512312578E-17));
#66273=CARTESIAN_POINT('',(-0.25,0.144337567297406,0.3));
#66274=CARTESIAN_POINT('',(1.76762539787485E-17,0.288675134594813,-5.55111512312578E-17));
#66275=CARTESIAN_POINT('Origin',(-0.25,-0.144337567297406,0.3));
#66276=CARTESIAN_POINT('',(-0.25,0.144337567297406,-5.55111512312578E-17));
#66277=CARTESIAN_POINT('Origin',(0.,0.,-5.55111512312578E-17));
#66278=CARTESIAN_POINT('Origin',(0.43,0.,-0.8));
#66279=CARTESIAN_POINT('',(-0.43,-5.26598123633362E-17,-0.8));
#66280=CARTESIAN_POINT('Origin',(0.,0.,-0.8));
#66281=CARTESIAN_POINT('Origin',(0.,0.,-0.765));
#66282=CARTESIAN_POINT('',(-0.465,-5.69460761603519E-17,-0.765));
#66283=CARTESIAN_POINT('Origin',(0.44,0.,-0.12));
#66284=CARTESIAN_POINT('',(-0.44,-5.38844591624835E-17,-0.12));
#66285=CARTESIAN_POINT('Origin',(0.,0.,-0.12));
#66286=CARTESIAN_POINT('Origin',(0.,0.,-0.12));
#66287=CARTESIAN_POINT('Origin',(0.,0.,-0.06));
#66288=CARTESIAN_POINT('',(-0.44,-5.38844591624836E-17,6.93889390390723E-18));
#66289=CARTESIAN_POINT('Origin',(0.,0.,0.));
#66290=CARTESIAN_POINT('',(-0.44,-5.38844591624835E-17,-0.06));
#66291=CARTESIAN_POINT('Origin',(0.68,0.,0.));
#66292=CARTESIAN_POINT('',(-0.68,-8.327598234202E-17,-1.73472347597681E-18));
#66293=CARTESIAN_POINT('Origin',(0.,0.,0.));
#66294=CARTESIAN_POINT('Origin',(0.,0.,0.01));
#66295=CARTESIAN_POINT('',(-0.7,-8.57252759403147E-17,0.02));
#66296=CARTESIAN_POINT('Origin',(0.,0.,0.02));
#66297=CARTESIAN_POINT('',(-0.69,-8.45006291411674E-17,0.01));
#66298=CARTESIAN_POINT('Origin',(0.,0.,0.14));
#66299=CARTESIAN_POINT('',(-0.7,-8.57252759403147E-17,0.26));
#66300=CARTESIAN_POINT('Origin',(0.,0.,0.26));
#66301=CARTESIAN_POINT('',(-0.7,-8.57252759403147E-17,0.14));
#66302=CARTESIAN_POINT('Origin',(0.,0.,0.28));
#66303=CARTESIAN_POINT('',(-0.66,-8.08266887437253E-17,0.3));
#66304=CARTESIAN_POINT('',(-0.68,8.327598234202E-17,0.28));
#66305=CARTESIAN_POINT('Origin',(0.,0.,0.3));
#66306=CARTESIAN_POINT('Origin',(0.,0.,0.3));
#86399=UNCERTAINTY_MEASURE_WITH_UNIT(LENGTH_MEASURE(0.001),#86430,
'DISTANCE_ACCURACY_VALUE',
'Maximum model space distance between geometric entities at asserted c
onnectivities');
#86409=UNCERTAINTY_MEASURE_WITH_UNIT(LENGTH_MEASURE(0.001),#86430,
'DISTANCE_ACCURACY_VALUE',
'Maximum model space distance between geometric entities at asserted c
onnectivities');
#86419=(
GEOMETRIC_REPRESENTATION_CONTEXT(3)
GLOBAL_UNCERTAINTY_ASSIGNED_CONTEXT((#86399))
GLOBAL_UNIT_ASSIGNED_CONTEXT((#86430,#86432,#86433))
REPRESENTATION_CONTEXT('','3D')
);
#86429=(
GEOMETRIC_REPRESENTATION_CONTEXT(3)
GLOBAL_UNCERTAINTY_ASSIGNED_CONTEXT((#86409))
GLOBAL_UNIT_ASSIGNED_CONTEXT((#86430,#86432,#86433))
REPRESENTATION_CONTEXT('','3D')
);
#86430=(
LENGTH_UNIT()
NAMED_UNIT(*)
SI_UNIT(.CENTI.,.METRE.)
);
#86432=(
NAMED_UNIT(*)
PLANE_ANGLE_UNIT()
SI_UNIT($,.RADIAN.)
);
#86433=(
NAMED_UNIT(*)
SI_UNIT($,.STERADIAN.)
SOLID_ANGLE_UNIT()
);
#86443=SHAPE_DEFINITION_REPRESENTATION(#86462,#86510);
#86462=PRODUCT_DEFINITION_SHAPE('',$,#86530);
#86510=SHAPE_REPRESENTATION('',(#16902),#86419);
#86520=PRODUCT_DEFINITION_CONTEXT('part definition',#86579,'design');
#86530=PRODUCT_DEFINITION('DIN908 M10x1 Hex Drive Plug',
'DIN908 M10x1 Hex Drive Plug',#86549,#86520);
#86549=PRODUCT_DEFINITION_FORMATION('',$,#86590);
#86579=APPLICATION_CONTEXT(
'Core Data for Automotive Mechanical Design Process');
#86580=PRODUCT_CONTEXT('part definition',#86579,'mechanical');
#86590=PRODUCT('DIN908 M10x1 Hex Drive Plug',
'DIN908 M10x1 Hex Drive Plug',$,(#86580));
#86609=PRESENTATION_STYLE_ASSIGNMENT((#86627));
#86627=SURFACE_STYLE_USAGE(.BOTH.,#86645);
#86645=SURFACE_SIDE_STYLE('',(#86663));
#86663=SURFACE_STYLE_FILL_AREA(#86681);
#86681=FILL_AREA_STYLE('Opaque(199,203,208)',(#86699));
#86699=FILL_AREA_STYLE_COLOUR('Opaque(199,203,208)',#86717);
#86717=COLOUR_RGB('Opaque(199,203,208)', 0.31764706, 0.68627451, 0.89019608);
ENDSEC;
END-ISO-10303-21;
